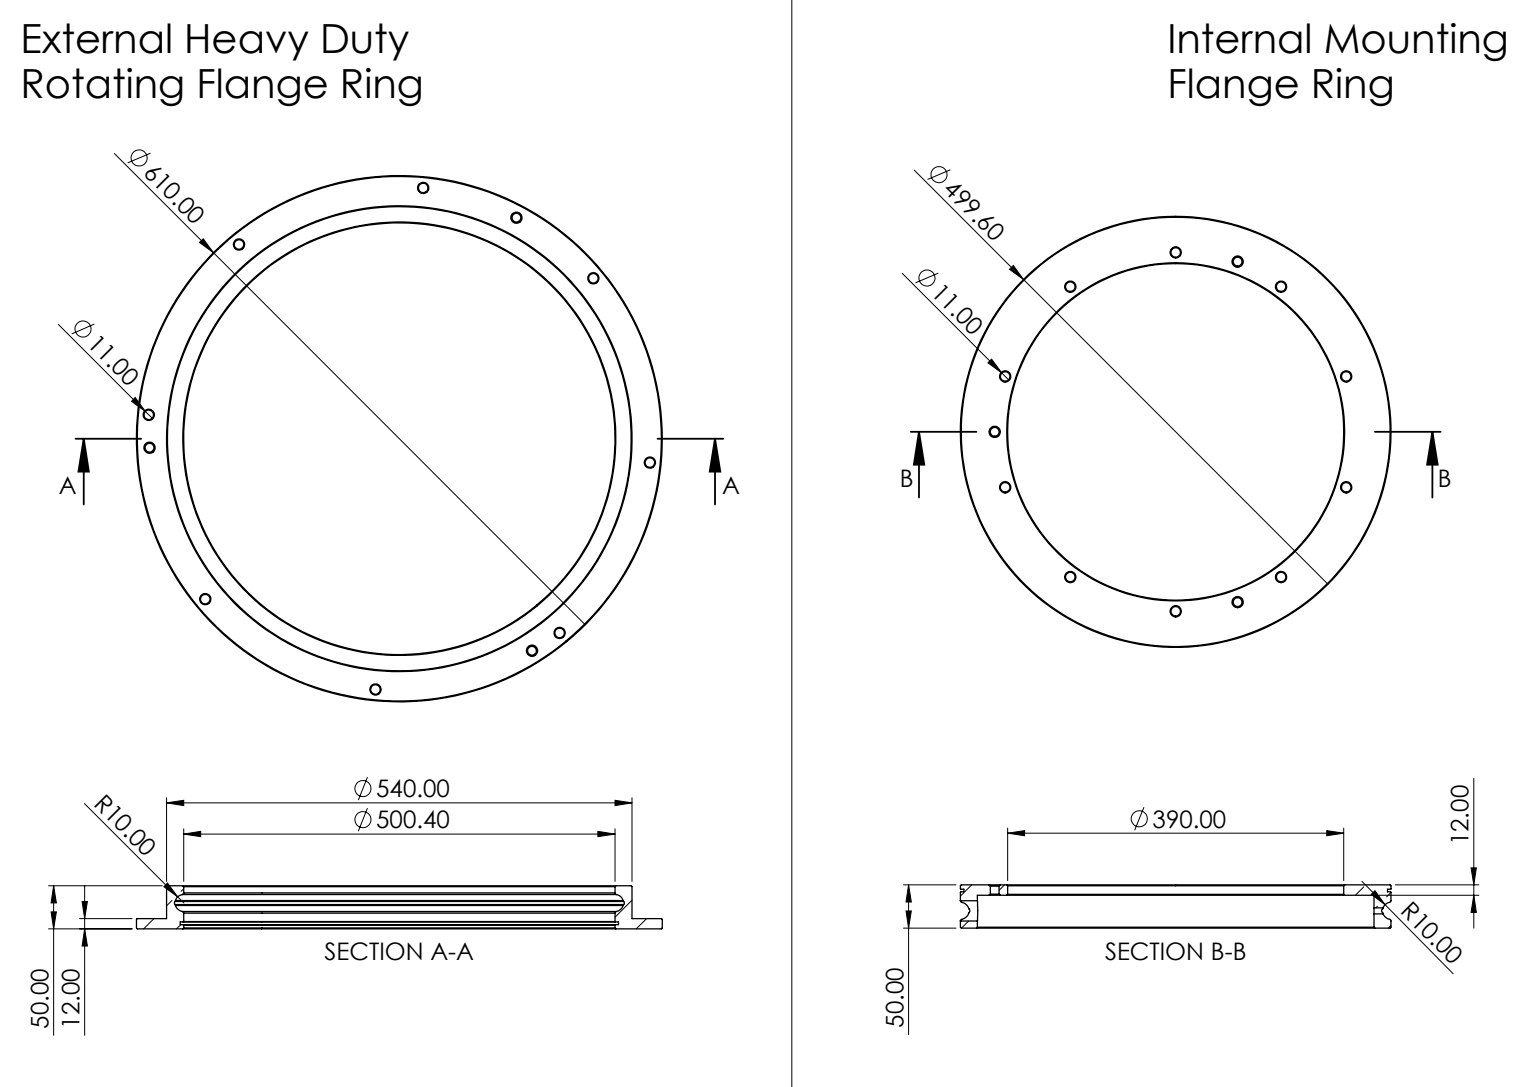
ISO-10303-21;
HEADER;
FILE_DESCRIPTION (('STEP AP214'),
    '1' );
FILE_NAME ('External Heavy Duty Rotating Flange Ring.step',
    '2026-10-09T12:49:55',
    ( '' ),
    ( '' ),
    'SwSTEP 2.0',
    'SolidWorks 2026',
    '' );
FILE_SCHEMA (( 'AUTOMOTIVE_DESIGN' ));
ENDSEC;

DATA;
#2=VECTOR ( 'NONE', #2010, 1000.000000000000000 ) ;
#15=DIRECTION ( 'NONE',  ( 0.6368676505102708330, 0.000000000000000000, 0.7709731485165535192 ) ) ;
#27=ORIENTED_EDGE ( 'NONE', *, *, #7436, .F. ) ;
#31=VECTOR ( 'NONE', #3967, 1000.000000000000000 ) ;
#39=EDGE_CURVE ( 'NONE', #10768, #6987, #12629, .T. ) ;
#40=AXIS2_PLACEMENT_3D ( 'NONE', #6246, #10297, #1175 ) ;
#41=ORIENTED_EDGE ( 'NONE', *, *, #3287, .F. ) ;
#42=EDGE_CURVE ( 'NONE', #9318, #6702, #6889, .T. ) ;
#55=ORIENTED_EDGE ( 'NONE', *, *, #3049, .F. ) ;
#57=CIRCLE ( 'NONE', #1754, 6.500000000000005329 ) ;
#60=CIRCLE ( 'NONE', #11338, 5.499999999999986677 ) ;
#64=DIRECTION ( 'NONE',  ( 0.6368676505102698338, 0.000000000000000000, 0.7709731485165541853 ) ) ;
#65=ORIENTED_EDGE ( 'NONE', *, *, #5983, .T. ) ;
#66=ADVANCED_FACE ( 'NONE', ( #7091 ), #10088, .F. ) ;
#75=CIRCLE ( 'NONE', #5391, 251.1999999999999886 ) ;
#77=AXIS2_PLACEMENT_3D ( 'NONE', #6499, #10557, #9543 ) ;
#79=ORIENTED_EDGE ( 'NONE', *, *, #10538, .F. ) ;
#83=DIRECTION ( 'NONE',  ( -0.000000000000000000, -1.000000000000000000, 0.000000000000000000 ) ) ;
#86=CARTESIAN_POINT ( 'NONE',  ( -182.4625818711933221, -29.00000000000000000, -220.8838070499919297 ) ) ;
#92=EDGE_CURVE ( 'NONE', #10082, #1949, #2942, .T. ) ;
#93=DIRECTION ( 'NONE',  ( 0.000000000000000000, 1.000000000000000000, 0.000000000000000000 ) ) ;
#94=ORIENTED_EDGE ( 'NONE', *, *, #12232, .T. ) ;
#95=ORIENTED_EDGE ( 'NONE', *, *, #11589, .F. ) ;
#96=CONICAL_SURFACE ( 'NONE', #12225, 250.1999999999999602, 0.7853981633975041232 ) ;
#100=CARTESIAN_POINT ( 'NONE',  ( -294.8238222686197787, -18.00000000000000000, -32.70078231947154279 ) ) ;
#104=AXIS2_PLACEMENT_3D ( 'NONE', #9793, #603, #2593 ) ;
#110=ORIENTED_EDGE ( 'NONE', *, *, #7597, .T. ) ;
#112=CIRCLE ( 'NONE', #2851, 5.500000000000007994 ) ;
#113=CARTESIAN_POINT ( 'NONE',  ( 229.2637990951503753, -30.00000000000000000, -180.9540284836414514 ) ) ;
#118=DIRECTION ( 'NONE',  ( -0.000000000000000000, -1.000000000000000000, 0.000000000000000000 ) ) ;
#124=DIRECTION ( 'NONE',  ( -0.6368676505102700558, 0.000000000000000000, -0.7709731485165541853 ) ) ;
#125=AXIS2_PLACEMENT_3D ( 'NONE', #10456, #7067, #12062 ) ;
#128=FACE_OUTER_BOUND ( 'NONE', #4868, .T. ) ;
#140=EDGE_CURVE ( 'NONE', #10237, #12935, #11247, .T. ) ;
#142=CARTESIAN_POINT ( 'NONE',  ( -27.68945685411286561, -30.00000000000000000, 290.6841825403027997 ) ) ;
#148=CARTESIAN_POINT ( 'NONE',  ( -185.9653539489998195, -30.00000000000000000, -225.1241593668329699 ) ) ;
#161=EDGE_CURVE ( 'NONE', #12208, #12419, #5216, .T. ) ;
#169=VERTEX_POINT ( 'NONE', #4404 ) ;
#177=ADVANCED_FACE ( 'NONE', ( #3475, #8488, #10550, #7486, #12547, #4470, #3403, #10415, #12679, #11557, #2351, #9424, #1290 ), #8427, .F. ) ;
#187=DIRECTION ( 'NONE',  ( 0.6368676505102709440, 0.000000000000000000, 0.7709731485165532971 ) ) ;
#195=CARTESIAN_POINT ( 'NONE',  ( -159.9811538081800393, -30.00000000000000000, -193.6684549073582389 ) ) ;
#206=DIRECTION ( 'NONE',  ( 0.6368676505102707219, 0.000000000000000000, 0.7709731485165535192 ) ) ;
#217=AXIS2_PLACEMENT_3D ( 'NONE', #2589, #10592, #3388 ) ;
#222=ORIENTED_EDGE ( 'NONE', *, *, #3793, .T. ) ;
#226=LINE ( 'NONE', #5219, #2394 ) ;
#230=ORIENTED_EDGE ( 'NONE', *, *, #4416, .F. ) ;
#232=ORIENTED_EDGE ( 'NONE', *, *, #7024, .T. ) ;
#233=CARTESIAN_POINT ( 'NONE',  ( 135.8846079354933352, -18.00000000000000000, -256.1940150085812888 ) ) ;
#235=ORIENTED_EDGE ( 'NONE', *, *, #8600, .T. ) ;
#237=VERTEX_POINT ( 'NONE', #3498 ) ;
#239=CARTESIAN_POINT ( 'NONE',  ( -171.9542656377731475, 19.00000000000000000, -208.1627500994694344 ) ) ;
#245=ORIENTED_EDGE ( 'NONE', *, *, #2691, .F. ) ;
#250=DIRECTION ( 'NONE',  ( -0.6368676505102706109, 0.000000000000000000, -0.7709731485165535192 ) ) ;
#251=DIRECTION ( 'NONE',  ( -0.000000000000000000, -1.000000000000000000, 0.000000000000000000 ) ) ;
#253=EDGE_CURVE ( 'NONE', #823, #11992, #3550, .T. ) ;
#266=FACE_OUTER_BOUND ( 'NONE', #2939, .T. ) ;
#268=CONICAL_SURFACE ( 'NONE', #4306, 251.1999999999999886, 0.7853981633974207455 ) ;
#272=CONICAL_SURFACE ( 'NONE', #12608, 6.500000000000005329, 0.7853981633974617127 ) ;
#276=ADVANCED_FACE ( 'NONE', ( #8553 ), #7175, .F. ) ;
#279=CARTESIAN_POINT ( 'NONE',  ( -159.2169126275676945, -3.061616997868385015E-14, -192.7432871291383663 ) ) ;
#282=CARTESIAN_POINT ( 'NONE',  ( 161.8917567597108018, -25.00000000000000000, 195.9813743529078920 ) ) ;
#284=EDGE_LOOP ( 'NONE', ( #11200, #1188, #5610, #7256 ) ) ;
#285=AXIS2_PLACEMENT_3D ( 'NONE', #10507, #6446, #1378 ) ;
#290=CARTESIAN_POINT ( 'NONE',  ( 0.000000000000000000, 2.772967769358929857, 0.000000000000000000 ) ) ;
#291=DIRECTION ( 'NONE',  ( -0.000000000000000000, -1.000000000000000000, 0.000000000000000000 ) ) ;
#294=CIRCLE ( 'NONE', #504, 5.500000000000015099 ) ;
#318=DIRECTION ( 'NONE',  ( 0.6368676505102716101, 0.000000000000000000, 0.7709731485165527420 ) ) ;
#321=DIRECTION ( 'NONE',  ( 0.000000000000000000, 1.000000000000000000, 0.000000000000000000 ) ) ;
#322=ORIENTED_EDGE ( 'NONE', *, *, #332, .F. ) ;
#327=VERTEX_POINT ( 'NONE', #7610 ) ;
#332=EDGE_CURVE ( 'NONE', #5214, #8298, #11654, .T. ) ;
#352=CARTESIAN_POINT ( 'NONE',  ( -171.9542656377731475, -18.00000000000000000, -208.1627500994694344 ) ) ;
#353=EDGE_LOOP ( 'NONE', ( #11784, #3307 ) ) ;
#354=VERTEX_POINT ( 'NONE', #3337 ) ;
#355=EDGE_CURVE ( 'NONE', #8227, #8752, #1859, .T. ) ;
#357=CARTESIAN_POINT ( 'NONE',  ( 235.1468102975488250, -18.00000000000000000, -194.2446334056325554 ) ) ;
#366=VERTEX_POINT ( 'NONE', #1547 ) ;
#367=DIRECTION ( 'NONE',  ( -0.6368676505102707219, 0.000000000000000000, -0.7709731485165535192 ) ) ;
#372=LINE ( 'NONE', #9371, #6679 ) ;
#373=CARTESIAN_POINT ( 'NONE',  ( 221.6213872890270977, -19.00000000000000000, -190.2057062658400923 ) ) ;
#377=CYLINDRICAL_SURFACE ( 'NONE', #4954, 5.100000000000003197 ) ;
#380=DIRECTION ( 'NONE',  ( -0.000000000000000000, -1.000000000000000000, 0.000000000000000000 ) ) ;
#383=DIRECTION ( 'NONE',  ( 0.6368676505102707219, 0.000000000000000000, 0.7709731485165536302 ) ) ;
#385=ADVANCED_FACE ( 'NONE', ( #12734 ), #10286, .F. ) ;
#392=CARTESIAN_POINT ( 'NONE',  ( -166.5596220099214690, -3.327561323230905366, -201.6321540179175713 ) ) ;
#401=ORIENTED_EDGE ( 'NONE', *, *, #140, .T. ) ;
#403=DIRECTION ( 'NONE',  ( 0.7709731485165535192, -0.000000000000000000, -0.6368676505102707219 ) ) ;
#410=DIRECTION ( 'NONE',  ( 0.6368676505102707219, 0.000000000000000000, 0.7709731485165535192 ) ) ;
#413=AXIS2_PLACEMENT_3D ( 'NONE', #9466, #8658, #6404 ) ;
#415=EDGE_LOOP ( 'NONE', ( #4979, #4482 ) ) ;
#418=ADVANCED_FACE ( 'NONE', ( #10744, #4871, #681, #11821, #9730, #1615, #2543, #12876, #6620, #1747, #10675, #555, #13009 ), #3605, .F. ) ;
#419=VECTOR ( 'NONE', #10160, 1000.000000000000000 ) ;
#424=FACE_OUTER_BOUND ( 'NONE', #2937, .T. ) ;
#427=CARTESIAN_POINT ( 'NONE',  ( -286.5445428119863323, -30.00000000000000000, -22.67813138875635204 ) ) ;
#435=DIRECTION ( 'NONE',  ( -0.000000000000000000, -1.000000000000000000, 0.000000000000000000 ) ) ;
#438=CARTESIAN_POINT ( 'NONE',  ( 171.9542656377731191, 19.00000000000000000, 208.1627500994694628 ) ) ;
#445=ADVANCED_FACE ( 'NONE', ( #12807 ), #6891, .F. ) ;
#446=EDGE_CURVE ( 'NONE', #12435, #9116, #11362, .T. ) ;
#449=ORIENTED_EDGE ( 'NONE', *, *, #355, .T. ) ;
#450=DIRECTION ( 'NONE',  ( 0.000000000000000000, 1.000000000000000000, 0.000000000000000000 ) ) ;
#452=CARTESIAN_POINT ( 'NONE',  ( -31.19222893191933821, -29.00000000000000000, 286.4438302234618163 ) ) ;
#454=CARTESIAN_POINT ( 'NONE',  ( 182.4625818711949137, -29.00000000000000000, 220.8838070499906507 ) ) ;
#455=PLANE ( 'NONE',  #2846 ) ;
#461=DIRECTION ( 'NONE',  ( 0.4503334343941581830, -0.7071067811865450192, 0.5451603414288000993 ) ) ;
#471=FACE_OUTER_BOUND ( 'NONE', #1035, .T. ) ;
#472=APPLICATION_CONTEXT ( 'automotive_design' ) ;
#481=AXIS2_PLACEMENT_3D ( 'NONE', #1897, #9541, #12361 ) ;
#484=AXIS2_PLACEMENT_3D ( 'NONE', #2681, #9957, #3755 ) ;
#500=DIRECTION ( 'NONE',  ( -0.6368676505102737195, 0.000000000000000000, -0.7709731485165509657 ) ) ;
#504=AXIS2_PLACEMENT_3D ( 'NONE', #4431, #380, #12767 ) ;
#507=DIRECTION ( 'NONE',  ( -0.000000000000000000, -1.000000000000000000, 0.000000000000000000 ) ) ;
#509=CARTESIAN_POINT ( 'NONE',  ( 185.9653539490014111, -30.00000000000000000, 225.1241593668316625 ) ) ;
#511=FACE_OUTER_BOUND ( 'NONE', #4843, .T. ) ;
#512=EDGE_CURVE ( 'NONE', #4498, #11239, #1570, .T. ) ;
#514=ORIENTED_EDGE ( 'NONE', *, *, #864, .T. ) ;
#518=CARTESIAN_POINT ( 'NONE',  ( 159.3442861576696998, -25.50000000000000000, 192.8974817588417352 ) ) ;
#526=DIRECTION ( 'NONE',  ( -0.6368676505102698338, 0.000000000000000000, -0.7709731485165541853 ) ) ;
#531=ORIENTED_EDGE ( 'NONE', *, *, #1101, .F. ) ;
#535=EDGE_CURVE ( 'NONE', #8515, #6953, #11631, .T. ) ;
#538=CARTESIAN_POINT ( 'NONE',  ( -290.6841825403030839, -19.00000000000000000, -27.68945685411394919 ) ) ;
#539=CARTESIAN_POINT ( 'NONE',  ( 27.68945685411497593, -19.00000000000000000, -290.6841825403026291 ) ) ;
#549=AXIS2_PLACEMENT_3D ( 'NONE', #4500, #3705, #6585 ) ;
#555=FACE_BOUND ( 'NONE', #1673, .T. ) ;
#557=CIRCLE ( 'NONE', #5230, 250.7000000000000171 ) ;
#558=DIRECTION ( 'NONE',  ( 0.6368676505102737195, 0.000000000000000000, 0.7709731485165509657 ) ) ;
#561=CARTESIAN_POINT ( 'NONE',  ( 182.4625818711949137, -19.00000000000000000, 220.8838070499906223 ) ) ;
#562=ORIENTED_EDGE ( 'NONE', *, *, #6556, .F. ) ;
#564=VERTEX_POINT ( 'NONE', #6140 ) ;
#565=CYLINDRICAL_SURFACE ( 'NONE', #12328, 254.1999999999999886 ) ;
#566=ORIENTED_EDGE ( 'NONE', *, *, #6725, .F. ) ;
#567=ORIENTED_EDGE ( 'NONE', *, *, #4107, .F. ) ;
#571=DIRECTION ( 'NONE',  ( -0.000000000000000000, -1.000000000000000000, 0.000000000000000000 ) ) ;
#577=ORIENTED_EDGE ( 'NONE', *, *, #3546, .T. ) ;
#581=DIRECTION ( 'NONE',  ( -0.000000000000000000, -1.000000000000000000, 0.000000000000000000 ) ) ;
#591=CARTESIAN_POINT ( 'NONE',  ( -0.000000000000000000, -3.165711975795909891E-14, 0.000000000000000000 ) ) ;
#592=ORIENTED_EDGE ( 'NONE', *, *, #10942, .T. ) ;
#598=DIRECTION ( 'NONE',  ( -0.000000000000000000, -1.000000000000000000, 0.000000000000000000 ) ) ;
#599=CARTESIAN_POINT ( 'NONE',  ( -0.000000000000000000, -11.79660968244695951, 0.000000000000000000 ) ) ;
#600=DIRECTION ( 'NONE',  ( -0.000000000000000000, -1.000000000000000000, 0.000000000000000000 ) ) ;
#603=DIRECTION ( 'NONE',  ( -0.000000000000000000, -1.000000000000000000, 0.000000000000000000 ) ) ;
#604=AXIS2_PLACEMENT_3D ( 'NONE', #8620, #4664, #3604 ) ;
#607=EDGE_CURVE ( 'NONE', #4062, #10624, #1004, .T. ) ;
#613=DIRECTION ( 'NONE',  ( -0.7709731485165535192, 0.000000000000000000, 0.6368676505102708330 ) ) ;
#614=AXIS2_PLACEMENT_3D ( 'NONE', #8258, #6261, #383 ) ;
#616=VECTOR ( 'NONE', #8753, 1000.000000000000000 ) ;
#619=DIRECTION ( 'NONE',  ( -0.6368676505102706109, 0.000000000000000000, -0.7709731485165535192 ) ) ;
#626=AXIS2_PLACEMENT_3D ( 'NONE', #7112, #7979, #4970 ) ;
#631=ORIENTED_EDGE ( 'NONE', *, *, #8325, .T. ) ;
#633=CARTESIAN_POINT ( 'NONE',  ( 140.0242476638101152, -30.00000000000000000, -251.1826895432237166 ) ) ;
#637=CARTESIAN_POINT ( 'NONE',  ( -27.68945685411286561, -30.00000000000000000, 290.6841825403027997 ) ) ;
#639=CIRCLE ( 'NONE', #9812, 5.100000000000003197 ) ;
#648=DIRECTION ( 'NONE',  ( 0.6368676505102716101, 0.000000000000000000, 0.7709731485165527420 ) ) ;
#656=DIRECTION ( 'NONE',  ( -0.4503334343941582940, -0.7071067811865450192, -0.5451603414288000993 ) ) ;
#660=ORIENTED_EDGE ( 'NONE', *, *, #9431, .T. ) ;
#663=EDGE_LOOP ( 'NONE', ( #7219, #7167, #8642, #12298 ) ) ;
#666=DIRECTION ( 'NONE',  ( -0.4503334343941627904, -0.7071067811865381358, -0.5451603414288054283 ) ) ;
#667=CARTESIAN_POINT ( 'NONE',  ( -287.1814104624966149, -19.00000000000000000, -23.44910453727290189 ) ) ;
#668=CARTESIAN_POINT ( 'NONE',  ( 0.000000000000000000, 0.000000000000000000, 0.000000000000000000 ) ) ;
#670=CARTESIAN_POINT ( 'NONE',  ( -229.2637990951503753, -18.00000000000000000, 180.9540284836414514 ) ) ;
#673=VECTOR ( 'NONE', #3157, 1000.000000000000000 ) ;
#676=ORIENTED_EDGE ( 'NONE', *, *, #6226, .T. ) ;
#679=ORIENTED_EDGE ( 'NONE', *, *, #4416, .T. ) ;
#681=FACE_BOUND ( 'NONE', #2232, .T. ) ;
#685=DIRECTION ( 'NONE',  ( 0.000000000000000000, 1.000000000000000000, 0.000000000000000000 ) ) ;
#688=AXIS2_PLACEMENT_3D ( 'NONE', #9443, #1239, #11509 ) ;
#689=CARTESIAN_POINT ( 'NONE',  ( -290.6841825403030839, -30.00000000000000000, -27.68945685411394919 ) ) ;
#695=EDGE_LOOP ( 'NONE', ( #12036, #7828, #9009, #10772 ) ) ;
#702=ADVANCED_FACE ( 'NONE', ( #4135 ), #8217, .F. ) ;
#706=LINE ( 'NONE', #8639, #7975 ) ;
#708=EDGE_CURVE ( 'NONE', #3236, #5526, #10611, .T. ) ;
#710=CARTESIAN_POINT ( 'NONE',  ( -27.68945685411286561, -19.00000000000000000, 290.6841825403027997 ) ) ;
#711=VECTOR ( 'NONE', #2929, 1000.000000000000000 ) ;
#712=ORIENTED_EDGE ( 'NONE', *, *, #12259, .T. ) ;
#715=ORIENTED_EDGE ( 'NONE', *, *, #5260, .T. ) ;
#718=CARTESIAN_POINT ( 'NONE',  ( 31.82909658243173467, -30.00000000000000000, -285.6728570749450569 ) ) ;
#720=AXIS2_PLACEMENT_3D ( 'NONE', #12565, #1304, #3418 ) ;
#727=ORIENTED_EDGE ( 'NONE', *, *, #5095, .T. ) ;
#736=FACE_OUTER_BOUND ( 'NONE', #11166, .T. ) ;
#741=AXIS2_PLACEMENT_3D ( 'NONE', #10234, #5164, #9243 ) ;
#750=ORIENTED_EDGE ( 'NONE', *, *, #4772, .F. ) ;
#752=CARTESIAN_POINT ( 'NONE',  ( -0.000000000000000000, -21.50000000000000000, 0.000000000000000000 ) ) ;
#753=CARTESIAN_POINT ( 'NONE',  ( -0.000000000000000000, -18.00000000000000000, 0.000000000000000000 ) ) ;
#757=CARTESIAN_POINT ( 'NONE',  ( 0.000000000000000000, 20.00000000000000000, 0.000000000000000000 ) ) ;
#761=COLOUR_RGB ( '', 0.72549020, 0.75294118, 0.79215686) ;
#764=CARTESIAN_POINT ( 'NONE',  ( 24.18668477630849267, -19.00000000000000000, -294.9245348571437262 ) ) ;
#767=CARTESIAN_POINT ( 'NONE',  ( -181.8257142206830679, -30.00000000000000000, -220.1128339014753692 ) ) ;
#779=VERTEX_POINT ( 'NONE', #9336 ) ;
#795=FACE_OUTER_BOUND ( 'NONE', #836, .T. ) ;
#805=AXIS2_PLACEMENT_3D ( 'NONE', #6711, #10765, #10635 ) ;
#814=DIRECTION ( 'NONE',  ( -0.000000000000000000, -1.000000000000000000, 0.000000000000000000 ) ) ;
#815=ORIENTED_EDGE ( 'NONE', *, *, #7409, .F. ) ;
#823=VERTEX_POINT ( 'NONE', #2331 ) ;
#830=DIRECTION ( 'NONE',  ( 0.6368676505102708330, 0.000000000000000000, 0.7709731485165535192 ) ) ;
#833=CARTESIAN_POINT ( 'NONE',  ( 0.000000000000000000, 20.00000000000000000, 0.000000000000000000 ) ) ;
#836=EDGE_LOOP ( 'NONE', ( #6634, #7940, #7084, #12038 ) ) ;
#837=FACE_OUTER_BOUND ( 'NONE', #10019, .T. ) ;
#855=CONICAL_SURFACE ( 'NONE', #12555, 6.500000000000005329, 0.7853981633974476129 ) ;
#856=ORIENTED_EDGE ( 'NONE', *, *, #12058, .F. ) ;
#857=ORIENTED_EDGE ( 'NONE', *, *, #9638, .T. ) ;
#859=ORIENTED_EDGE ( 'NONE', *, *, #3793, .F. ) ;
#862=CARTESIAN_POINT ( 'NONE',  ( -0.000000000000000000, -29.00000000000000000, 0.000000000000000000 ) ) ;
#864=EDGE_CURVE ( 'NONE', #6987, #11199, #7273, .T. ) ;
#873=ORIENTED_EDGE ( 'NONE', *, *, #8104, .T. ) ;
#877=CARTESIAN_POINT ( 'NONE',  ( -290.6841825403030839, -18.00000000000000000, -27.68945685411394919 ) ) ;
#886=ORIENTED_EDGE ( 'NONE', *, *, #7689, .F. ) ;
#890=ORIENTED_EDGE ( 'NONE', *, *, #10293, .T. ) ;
#891=DIRECTION ( 'NONE',  ( 0.6368676505102707219, 0.000000000000000000, 0.7709731485165535192 ) ) ;
#893=CARTESIAN_POINT ( 'NONE',  ( 160.6180214586902366, 11.79660968244693997, 194.4394280558747994 ) ) ;
#894=AXIS2_PLACEMENT_3D ( 'NONE', #1605, #600, #9791 ) ;
#895=EDGE_CURVE ( 'NONE', #6702, #6924, #4337, .T. ) ;
#900=VERTEX_POINT ( 'NONE', #8538 ) ;
#908=LINE ( 'NONE', #2961, #1944 ) ;
#910=DIRECTION ( 'NONE',  ( 0.6368676505102709440, 0.000000000000000000, 0.7709731485165532971 ) ) ;
#911=EDGE_CURVE ( 'NONE', #10031, #1416, #5411, .T. ) ;
#914=APPLICATION_CONTEXT ( 'automotive_design' ) ;
#919=UNCERTAINTY_MEASURE_WITH_UNIT (LENGTH_MEASURE( 1.000000000000000082E-05 ), #5049, 'distance_accuracy_value', 'NONE');
#920=ORIENTED_EDGE ( 'NONE', *, *, #11171, .T. ) ;
#927=VECTOR ( 'NONE', #6570, 1000.000000000000000 ) ;
#931=DIRECTION ( 'NONE',  ( 0.6368676505102707219, 0.000000000000000000, 0.7709731485165535192 ) ) ;
#935=SURFACE_STYLE_USAGE ( .BOTH. , #10063 ) ;
#941=VERTEX_POINT ( 'NONE', #11733 ) ;
#943=CARTESIAN_POINT ( 'NONE',  ( 286.5445428119865028, -30.00000000000000000, 22.67813138875427015 ) ) ;
#945=VECTOR ( 'NONE', #7892, 1000.000000000000000 ) ;
#949=DIRECTION ( 'NONE',  ( -0.000000000000000000, -1.000000000000000000, 0.000000000000000000 ) ) ;
#955=AXIS2_PLACEMENT_3D ( 'NONE', #9704, #11726, #9580 ) ;
#957=CARTESIAN_POINT ( 'NONE',  ( -289.8128292627096130, -30.00000000000000000, 10.41748504886635907 ) ) ;
#958=EDGE_LOOP ( 'NONE', ( #8262, #10296, #3960, #7089 ) ) ;
#959=ORIENTED_EDGE ( 'NONE', *, *, #1758, .F. ) ;
#960=CARTESIAN_POINT ( 'NONE',  ( -0.000000000000000000, -11.79660968244695951, 0.000000000000000000 ) ) ;
#965=DIRECTION ( 'NONE',  ( 0.4503334343941555740, 0.7071067811865490160, 0.5451603414287971017 ) ) ;
#969=ORIENTED_EDGE ( 'NONE', *, *, #5981, .F. ) ;
#971=ORIENTED_EDGE ( 'NONE', *, *, #6486, .F. ) ;
#975=DIRECTION ( 'NONE',  ( -0.6368676505102707219, 0.000000000000000000, -0.7709731485165535192 ) ) ;
#984=ORIENTED_EDGE ( 'NONE', *, *, #6119, .T. ) ;
#986=EDGE_CURVE ( 'NONE', #7844, #5825, #4648, .T. ) ;
#989=ORIENTED_EDGE ( 'NONE', *, *, #7409, .T. ) ;
#996=SURFACE_STYLE_FILL_AREA ( #11127 ) ;
#1004=LINE ( 'NONE', #4497, #7838 ) ;
#1005=PLANE ( 'NONE',  #8520 ) ;
#1018=ORIENTED_EDGE ( 'NONE', *, *, #10942, .F. ) ;
#1019=DIRECTION ( 'NONE',  ( 0.6368676505102707219, 0.000000000000000000, 0.7709731485165535192 ) ) ;
#1023=EDGE_CURVE ( 'NONE', #11697, #2079, #4230, .T. ) ;
#1027=ORIENTED_EDGE ( 'NONE', *, *, #1507, .T. ) ;
#1029=TOROIDAL_SURFACE ( 'NONE', #4427, 252.1999999999999886, 2.000000000000000000 ) ;
#1033=ORIENTED_EDGE ( 'NONE', *, *, #11937, .T. ) ;
#1035=EDGE_LOOP ( 'NONE', ( #566, #11162, #7813, #5039 ) ) ;
#1043=VECTOR ( 'NONE', #4814, 1000.000000000000000 ) ;
#1047=CIRCLE ( 'NONE', #6376, 251.1999999999999886 ) ;
#1061=CIRCLE ( 'NONE', #12129, 5.100000000000003197 ) ;
#1067=ORIENTED_EDGE ( 'NONE', *, *, #11182, .T. ) ;
#1075=CYLINDRICAL_SURFACE ( 'NONE', #11982, 5.500000000000007994 ) ;
#1077=VECTOR ( 'NONE', #1474, 1000.000000000000000 ) ;
#1079=ORIENTED_EDGE ( 'NONE', *, *, #1023, .T. ) ;
#1086=ADVANCED_FACE ( 'NONE', ( #736 ), #6375, .F. ) ;
#1092=DIRECTION ( 'NONE',  ( 0.6368676505102707219, 0.000000000000000000, 0.7709731485165535192 ) ) ;
#1095=ORIENTED_EDGE ( 'NONE', *, *, #10168, .F. ) ;
#1096=DIRECTION ( 'NONE',  ( -0.6368676505102707219, 0.000000000000000000, -0.7709731485165535192 ) ) ;
#1100=VERTEX_POINT ( 'NONE', #2649 ) ;
#1101=EDGE_CURVE ( 'NONE', #10423, #5861, #4770, .T. ) ;
#1102=CARTESIAN_POINT ( 'NONE',  ( 225.1241593668336236, -30.00000000000000000, -185.9653539489990521 ) ) ;
#1105=CARTESIAN_POINT ( 'NONE',  ( -0.000000000000000000, -3.165711975795909891E-14, 0.000000000000000000 ) ) ;
#1107=DIRECTION ( 'NONE',  ( -0.000000000000000000, -1.000000000000000000, 0.000000000000000000 ) ) ;
#1108=DIRECTION ( 'NONE',  ( 0.6368676505102716101, 0.000000000000000000, 0.7709731485165527420 ) ) ;
#1109=ADVANCED_FACE ( 'NONE', ( #9059 ), #7125, .T. ) ;
#1114=ORIENTED_EDGE ( 'NONE', *, *, #42, .T. ) ;
#1115=DIRECTION ( 'NONE',  ( -0.000000000000000000, -1.000000000000000000, 0.000000000000000000 ) ) ;
#1119=FACE_OUTER_BOUND ( 'NONE', #12151, .T. ) ;
#1125=CARTESIAN_POINT ( 'NONE',  ( 185.9653539490014111, -19.00000000000000000, 225.1241593668316625 ) ) ;
#1127=AXIS2_PLACEMENT_3D ( 'NONE', #9176, #12175, #4106 ) ;
#1133=DIRECTION ( 'NONE',  ( 0.000000000000000000, 1.000000000000000000, 0.000000000000000000 ) ) ;
#1135=ORIENTED_EDGE ( 'NONE', *, *, #3577, .F. ) ;
#1137=ADVANCED_FACE ( 'NONE', ( #5929 ), #1377, .T. ) ;
#1144=VECTOR ( 'NONE', #5770, 1000.000000000000000 ) ;
#1154=ADVANCED_FACE ( 'NONE', ( #795 ), #2947, .T. ) ;
#1155=ORIENTED_EDGE ( 'NONE', *, *, #12673, .T. ) ;
#1156=EDGE_CURVE ( 'NONE', #12208, #9851, #8613, .T. ) ;
#1159=DIRECTION ( 'NONE',  ( -0.000000000000000000, -1.000000000000000000, 0.000000000000000000 ) ) ;
#1166=AXIS2_PLACEMENT_3D ( 'NONE', #11964, #2622, #4559 ) ;
#1170=VERTEX_POINT ( 'NONE', #8929 ) ;
#1175=DIRECTION ( 'NONE',  ( 0.6368676505102707219, 0.000000000000000000, 0.7709731485165535192 ) ) ;
#1187=CIRCLE ( 'NONE', #8225, 6.500000000000005329 ) ;
#1188=ORIENTED_EDGE ( 'NONE', *, *, #8602, .F. ) ;
#1189=VECTOR ( 'NONE', #11301, 1000.000000000000000 ) ;
#1193=ORIENTED_EDGE ( 'NONE', *, *, #6647, .T. ) ;
#1196=DIRECTION ( 'NONE',  ( 0.6368676505102707219, 0.000000000000000000, 0.7709731485165535192 ) ) ;
#1199=ADVANCED_FACE ( 'NONE', ( #6721 ), #10305, .F. ) ;
#1200=DIRECTION ( 'NONE',  ( 0.000000000000000000, 1.000000000000000000, 0.000000000000000000 ) ) ;
#1203=CARTESIAN_POINT ( 'NONE',  ( -289.8128292627096130, -19.40000000000000213, 10.41748504886635907 ) ) ;
#1208=FACE_OUTER_BOUND ( 'NONE', #353, .T. ) ;
#1216=DIRECTION ( 'NONE',  ( 0.000000000000000000, 1.000000000000000000, 0.000000000000000000 ) ) ;
#1221=DIRECTION ( 'NONE',  ( 0.6368676505102708330, 0.000000000000000000, 0.7709731485165535192 ) ) ;
#1224=CARTESIAN_POINT ( 'NONE',  ( -229.2637990951503753, -30.00000000000000000, 180.9540284836414514 ) ) ;
#1228=ADVANCED_FACE ( 'NONE', ( #7706, #1712 ), #455, .F. ) ;
#1231=ORIENTED_EDGE ( 'NONE', *, *, #3028, .T. ) ;
#1233=ORIENTED_EDGE ( 'NONE', *, *, #8587, .T. ) ;
#1234=ORIENTED_EDGE ( 'NONE', *, *, #895, .T. ) ;
#1236=CARTESIAN_POINT ( 'NONE',  ( -0.000000000000000000, -1.848645179577135034, 0.000000000000000000 ) ) ;
#1238=CARTESIAN_POINT ( 'NONE',  ( -225.1241593668336236, -18.00000000000000000, 185.9653539489990521 ) ) ;
#1239=DIRECTION ( 'NONE',  ( -0.000000000000000000, -1.000000000000000000, 0.000000000000000000 ) ) ;
#1240=CARTESIAN_POINT ( 'NONE',  ( 0.000000000000000000, 0.000000000000000000, 0.000000000000000000 ) ) ;
#1244=VERTEX_POINT ( 'NONE', #718 ) ;
#1247=DIRECTION ( 'NONE',  ( -0.000000000000000000, -1.000000000000000000, 0.000000000000000000 ) ) ;
#1250=ORIENTED_EDGE ( 'NONE', *, *, #5677, .T. ) ;
#1251=AXIS2_PLACEMENT_3D ( 'NONE', #9452, #3363, #11450 ) ;
#1252=EDGE_CURVE ( 'NONE', #10483, #10082, #3490, .T. ) ;
#1255=ADVANCED_FACE ( 'NONE', ( #10775 ), #11745, .F. ) ;
#1258=AXIS2_PLACEMENT_3D ( 'NONE', #12752, #3616, #7684 ) ;
#1265=AXIS2_PLACEMENT_3D ( 'NONE', #8906, #12976, #4769 ) ;
#1268=ORIENTED_EDGE ( 'NONE', *, *, #8533, .T. ) ;
#1272=DIRECTION ( 'NONE',  ( -0.4503334343941627904, -0.7071067811865381358, -0.5451603414288054283 ) ) ;
#1273=VECTOR ( 'NONE', #5631, 1000.000000000000000 ) ;
#1274=CARTESIAN_POINT ( 'NONE',  ( -289.8128292627096130, -30.00000000000000000, 10.41748504886635907 ) ) ;
#1280=CARTESIAN_POINT ( 'NONE',  ( 228.6269314446401211, -19.00000000000000000, -181.7250016321579835 ) ) ;
#1287=ORIENTED_EDGE ( 'NONE', *, *, #512, .T. ) ;
#1290=FACE_OUTER_BOUND ( 'NONE', #10006, .T. ) ;
#1293=DIRECTION ( 'NONE',  ( -0.6368676505102707219, 0.000000000000000000, -0.7709731485165536302 ) ) ;
#1300=FACE_OUTER_BOUND ( 'NONE', #2873, .T. ) ;
#1301=EDGE_LOOP ( 'NONE', ( #12296, #7141, #10815, #12253 ) ) ;
#1303=EDGE_CURVE ( 'NONE', #5861, #10423, #3419, .T. ) ;
#1304=DIRECTION ( 'NONE',  ( -0.000000000000000000, -1.000000000000000000, 0.000000000000000000 ) ) ;
#1307=CARTESIAN_POINT ( 'NONE',  ( -225.1241593668336236, -30.00000000000000000, 185.9653539489990521 ) ) ;
#1312=ORIENTED_EDGE ( 'NONE', *, *, #4894, .T. ) ;
#1314=CARTESIAN_POINT ( 'NONE',  ( 153.9282213272189495, -28.60000000000000142, 245.7765299597151341 ) ) ;
#1318=LINE ( 'NONE', #4501, #9779 ) ;
#1321=EDGE_CURVE ( 'NONE', #1858, #4661, #11845, .T. ) ;
#1325=CARTESIAN_POINT ( 'NONE',  ( 158.0678610555357295, -30.00000000000000000, 250.7878554250727632 ) ) ;
#1327=CARTESIAN_POINT ( 'NONE',  ( 0.000000000000000000, 20.00000000000000000, 0.000000000000000000 ) ) ;
#1333=EDGE_LOOP ( 'NONE', ( #4898, #4678 ) ) ;
#1342=CIRCLE ( 'NONE', #9629, 10.00000000000000178 ) ;
#1346=ADVANCED_FACE ( 'NONE', ( #6589 ), #8973, .F. ) ;
#1347=EDGE_LOOP ( 'NONE', ( #9668, #11883, #1234, #3830 ) ) ;
#1348=CIRCLE ( 'NONE', #1127, 10.00000000000000178 ) ;
#1352=ORIENTED_EDGE ( 'NONE', *, *, #7689, .T. ) ;
#1359=CARTESIAN_POINT ( 'NONE',  ( 153.9282213272189495, -30.00000000000000000, 245.7765299597151341 ) ) ;
#1372=CARTESIAN_POINT ( 'NONE',  ( 158.0678610555357295, -30.00000000000000000, 250.7878554250727632 ) ) ;
#1377=TOROIDAL_SURFACE ( 'NONE', #12236, 261.5294117647060261, 2.000000000000000000 ) ;
#1378=DIRECTION ( 'NONE',  ( -0.6368676505102698338, 0.000000000000000000, -0.7709731485165542964 ) ) ;
#1381=CARTESIAN_POINT ( 'NONE',  ( 185.9653539490014111, -30.00000000000000000, 225.1241593668316625 ) ) ;
#1384=CARTESIAN_POINT ( 'NONE',  ( 0.000000000000000000, 19.00000000000000000, 0.000000000000000000 ) ) ;
#1398=ADVANCED_FACE ( 'NONE', ( #1640 ), #3211, .F. ) ;
#1402=VECTOR ( 'NONE', #5824, 1000.000000000000114 ) ;
#1405=CYLINDRICAL_SURFACE ( 'NONE', #6256, 5.500000000000007994 ) ;
#1409=DIRECTION ( 'NONE',  ( -0.000000000000000000, -1.000000000000000000, 0.000000000000000000 ) ) ;
#1413=DIRECTION ( 'NONE',  ( -0.000000000000000000, -1.000000000000000000, 0.000000000000000000 ) ) ;
#1415=ORIENTED_EDGE ( 'NONE', *, *, #3005, .F. ) ;
#1416=VERTEX_POINT ( 'NONE', #11976 ) ;
#1429=AXIS2_PLACEMENT_3D ( 'NONE', #12612, #4348, #11623 ) ;
#1433=DIRECTION ( 'NONE',  ( -0.000000000000000000, -1.000000000000000000, 0.000000000000000000 ) ) ;
#1434=EDGE_CURVE ( 'NONE', #5762, #8072, #10667, .T. ) ;
#1437=CYLINDRICAL_SURFACE ( 'NONE', #7753, 270.0000000000000000 ) ;
#1447=DIRECTION ( 'NONE',  ( -0.000000000000000000, -1.000000000000000000, 0.000000000000000000 ) ) ;
#1452=DIRECTION ( 'NONE',  ( 0.6368676505102689456, 0.000000000000000000, 0.7709731485165549625 ) ) ;
#1456=AXIS2_PLACEMENT_3D ( 'NONE', #5382, #2248, #10445 ) ;
#1457=CONICAL_SURFACE ( 'NONE', #6578, 5.500000000000015099, 0.7853981633974461696 ) ;
#1461=AXIS2_PLACEMENT_3D ( 'NONE', #10142, #7221, #4277 ) ;
#1465=CARTESIAN_POINT ( 'NONE',  ( 225.1241593668336236, -30.00000000000000000, -185.9653539489990521 ) ) ;
#1474=DIRECTION ( 'NONE',  ( -0.000000000000000000, -1.000000000000000000, 0.000000000000000000 ) ) ;
#1494=ADVANCED_FACE ( 'NONE', ( #2962 ), #8547, .F. ) ;
#1495=CARTESIAN_POINT ( 'NONE',  ( -23.54981712579610331, -30.00000000000000000, 295.6955080056604288 ) ) ;
#1496=EDGE_LOOP ( 'NONE', ( #3668, #5704 ) ) ;
#1499=DIRECTION ( 'NONE',  ( -0.000000000000000000, -1.000000000000000000, 0.000000000000000000 ) ) ;
#1506=DIRECTION ( 'NONE',  ( 0.6368676505102716101, 0.000000000000000000, 0.7709731485165527420 ) ) ;
#1507=EDGE_CURVE ( 'NONE', #10768, #8072, #5850, .T. ) ;
#1516=DIRECTION ( 'NONE',  ( 0.000000000000000000, 1.000000000000000000, 0.000000000000000000 ) ) ;
#1520=AXIS2_PLACEMENT_3D ( 'NONE', #2880, #9030, #4018 ) ;
#1521=DIRECTION ( 'NONE',  ( 0.7709731485165535192, 0.000000000000000000, -0.6368676505102707219 ) ) ;
#1524=EDGE_CURVE ( 'NONE', #8945, #4077, #11104, .T. ) ;
#1526=ORIENTED_EDGE ( 'NONE', *, *, #4011, .F. ) ;
#1534=DIRECTION ( 'NONE',  ( 0.6368676505102707219, 0.000000000000000000, 0.7709731485165535192 ) ) ;
#1536=DIRECTION ( 'NONE',  ( -0.000000000000000000, -1.000000000000000000, 0.000000000000000000 ) ) ;
#1540=VECTOR ( 'NONE', #7162, 1000.000000000000000 ) ;
#1547=CARTESIAN_POINT ( 'NONE',  ( 171.3173979872628365, 20.00000000000000000, 207.3917769509529307 ) ) ;
#1555=DIRECTION ( 'NONE',  ( 0.000000000000000000, 1.000000000000000000, 0.000000000000000000 ) ) ;
#1561=FACE_OUTER_BOUND ( 'NONE', #6989, .T. ) ;
#1563=ORIENTED_EDGE ( 'NONE', *, *, #7436, .T. ) ;
#1569=CARTESIAN_POINT ( 'NONE',  ( -159.9811538081799824, 20.00000000000000000, -193.6684549073582389 ) ) ;
#1570=CIRCLE ( 'NONE', #9020, 2.000000000000000444 ) ;
#1573=DIRECTION ( 'NONE',  ( -0.000000000000000000, -1.000000000000000000, 0.000000000000000000 ) ) ;
#1579=ORIENTED_EDGE ( 'NONE', *, *, #8609, .T. ) ;
#1581=EDGE_LOOP ( 'NONE', ( #11025, #11383 ) ) ;
#1589=CARTESIAN_POINT ( 'NONE',  ( 294.1869546181097235, -19.00000000000000000, 31.92980917095290749 ) ) ;
#1594=ORIENTED_EDGE ( 'NONE', *, *, #9005, .T. ) ;
#1601=CARTESIAN_POINT ( 'NONE',  ( 185.9653539490014111, -19.00000000000000000, 225.1241593668316625 ) ) ;
#1605=CARTESIAN_POINT ( 'NONE',  ( 135.8846079354933352, -30.00000000000000000, -256.1940150085812888 ) ) ;
#1610=AXIS2_PLACEMENT_3D ( 'NONE', #2610, #1555, #11696 ) ;
#1613=EDGE_LOOP ( 'NONE', ( #1135, #1114, #5557, #3703 ) ) ;
#1615=FACE_BOUND ( 'NONE', #10482, .T. ) ;
#1619=FACE_OUTER_BOUND ( 'NONE', #958, .T. ) ;
#1621=DIRECTION ( 'NONE',  ( -0.000000000000000000, -1.000000000000000000, 0.000000000000000000 ) ) ;
#1633=ORIENTED_EDGE ( 'NONE', *, *, #8745, .F. ) ;
#1638=ORIENTED_EDGE ( 'NONE', *, *, #12741, .T. ) ;
#1639=CARTESIAN_POINT ( 'NONE',  ( -221.6213872890270977, -29.00000000000000000, 190.2057062658400923 ) ) ;
#1640=FACE_OUTER_BOUND ( 'NONE', #10969, .T. ) ;
#1641=DIRECTION ( 'NONE',  ( -0.000000000000000000, -1.000000000000000000, 0.000000000000000000 ) ) ;
#1651=EDGE_LOOP ( 'NONE', ( #9963, #7430, #3042, #2675 ) ) ;
#1652=ADVANCED_FACE ( 'NONE', ( #9945, #11211 ), #2077, .F. ) ;
#1659=DIRECTION ( 'NONE',  ( 0.6368676505102716101, 0.000000000000000000, 0.7709731485165527420 ) ) ;
#1661=DIRECTION ( 'NONE',  ( -0.4503334343941627904, -0.7071067811865381358, -0.5451603414288054283 ) ) ;
#1662=CARTESIAN_POINT ( 'NONE',  ( -290.6841825403030839, -30.00000000000000000, -27.68945685411394919 ) ) ;
#1672=ORIENTED_EDGE ( 'NONE', *, *, #4894, .F. ) ;
#1673=EDGE_LOOP ( 'NONE', ( #4388, #2858 ) ) ;
#1675=DIRECTION ( 'NONE',  ( 0.000000000000000000, 1.000000000000000000, 0.000000000000000000 ) ) ;
#1679=AXIS2_PLACEMENT_3D ( 'NONE', #1125, #8059, #931 ) ;
#1680=CIRCLE ( 'NONE', #1258, 2.500000000000025313 ) ;
#1689=AXIS2_PLACEMENT_3D ( 'NONE', #11529, #5578, #3440 ) ;
#1692=ORIENTED_EDGE ( 'NONE', *, *, #2881, .T. ) ;
#1709=CIRCLE ( 'NONE', #4673, 5.500000000000015099 ) ;
#1712=FACE_OUTER_BOUND ( 'NONE', #7058, .T. ) ;
#1719=ORIENTED_EDGE ( 'NONE', *, *, #9961, .T. ) ;
#1722=ORIENTED_EDGE ( 'NONE', *, *, #12793, .T. ) ;
#1723=EDGE_CURVE ( 'NONE', #11697, #10031, #10016, .T. ) ;
#1725=VERTEX_POINT ( 'NONE', #1951 ) ;
#1730=DIRECTION ( 'NONE',  ( -0.000000000000000000, -1.000000000000000000, 0.000000000000000000 ) ) ;
#1734=DIRECTION ( 'NONE',  ( -0.6368676505102698338, 0.000000000000000000, -0.7709731485165541853 ) ) ;
#1736=DIRECTION ( 'NONE',  ( 0.4503334343941626794, -0.7071067811865380248, 0.5451603414288055394 ) ) ;
#1745=EDGE_LOOP ( 'NONE', ( #4372, #10086 ) ) ;
#1747=FACE_BOUND ( 'NONE', #7385, .T. ) ;
#1748=ADVANCED_FACE ( 'NONE', ( #12150 ), #12548, .T. ) ;
#1751=DIRECTION ( 'NONE',  ( 0.6368676505102716101, 0.000000000000000000, 0.7709731485165527420 ) ) ;
#1754=AXIS2_PLACEMENT_3D ( 'NONE', #1307, #8638, #7507 ) ;
#1755=CARTESIAN_POINT ( 'NONE',  ( -286.5648042451072115, -19.40000000000000213, 14.34944810630078393 ) ) ;
#1758=EDGE_CURVE ( 'NONE', #169, #11069, #11704, .T. ) ;
#1761=ORIENTED_EDGE ( 'NONE', *, *, #11687, .T. ) ;
#1763=ORIENTED_EDGE ( 'NONE', *, *, #9005, .F. ) ;
#1765=CIRCLE ( 'NONE', #11335, 250.1999999999999602 ) ;
#1771=( NAMED_UNIT ( * ) SI_UNIT ( $, .STERADIAN. ) SOLID_ANGLE_UNIT ( ) );
#1772=DIRECTION ( 'NONE',  ( 0.4503334343941562956, -0.7071067811865480168, 0.5451603414287978788 ) ) ;
#1775=CIRCLE ( 'NONE', #4735, 2.000000000000000444 ) ;
#1777=VECTOR ( 'NONE', #3678, 1000.000000000000000 ) ;
#1779=ORIENTED_EDGE ( 'NONE', *, *, #1434, .F. ) ;
#1781=AXIS2_PLACEMENT_3D ( 'NONE', #3671, #5814, #5882 ) ;
#1785=AXIS2_PLACEMENT_3D ( 'NONE', #3701, #10704, #8643 ) ;
#1794=AXIS2_PLACEMENT_3D ( 'NONE', #8969, #7970, #1096 ) ;
#1795=ORIENTED_EDGE ( 'NONE', *, *, #8602, .T. ) ;
#1801=AXIS2_PLACEMENT_3D ( 'NONE', #3853, #3046, #7061 ) ;
#1803=ADVANCED_FACE ( 'NONE', ( #9351 ), #6808, .F. ) ;
#1807=AXIS2_PLACEMENT_3D ( 'NONE', #10386, #9396, #11401 ) ;
#1816=CARTESIAN_POINT ( 'NONE',  ( 192.8974817588416784, -30.00000000000000000, -159.3442861576696998 ) ) ;
#1820=CYLINDRICAL_SURFACE ( 'NONE', #1832, 250.1999999999999602 ) ;
#1827=EDGE_LOOP ( 'NONE', ( #6840, #4915 ) ) ;
#1828=EDGE_CURVE ( 'NONE', #6569, #4077, #6592, .T. ) ;
#1832=AXIS2_PLACEMENT_3D ( 'NONE', #5888, #814, #4877 ) ;
#1841=EDGE_LOOP ( 'NONE', ( #2251, #12872 ) ) ;
#1848=FACE_OUTER_BOUND ( 'NONE', #8984, .T. ) ;
#1855=EDGE_LOOP ( 'NONE', ( #6438, #8683, #1233, #4846 ) ) ;
#1858=VERTEX_POINT ( 'NONE', #6222 ) ;
#1859=CIRCLE ( 'NONE', #10578, 5.500000000000015099 ) ;
#1865=DIRECTION ( 'NONE',  ( -0.4503334343941556295, 0.7071067811865489050, -0.5451603414287969906 ) ) ;
#1866=AXIS2_PLACEMENT_3D ( 'NONE', #7709, #5710, #9769 ) ;
#1869=DIRECTION ( 'NONE',  ( 0.6368676505102696117, 0.000000000000000000, 0.7709731485165545184 ) ) ;
#1871=CARTESIAN_POINT ( 'NONE',  ( -160.3845033201291130, -9.830508068730530624, -194.1567379013694392 ) ) ;
#1875=CARTESIAN_POINT ( 'NONE',  ( -0.000000000000000000, -19.00000000000000000, 0.000000000000000000 ) ) ;
#1888=AXIS2_PLACEMENT_3D ( 'NONE', #9686, #2619, #830 ) ;
#1889=ORIENTED_EDGE ( 'NONE', *, *, #7552, .T. ) ;
#1892=ORIENTED_EDGE ( 'NONE', *, *, #10963, .T. ) ;
#1897=CARTESIAN_POINT ( 'NONE',  ( -0.000000000000000000, -29.00000000000000000, 0.000000000000000000 ) ) ;
#1900=AXIS2_PLACEMENT_3D ( 'NONE', #7905, #11788, #10776 ) ;
#1911=FACE_OUTER_BOUND ( 'NONE', #7471, .T. ) ;
#1913=LINE ( 'NONE', #4039, #11378 ) ;
#1921=VERTEX_POINT ( 'NONE', #4462 ) ;
#1923=ORIENTED_EDGE ( 'NONE', *, *, #3172, .F. ) ;
#1933=EDGE_CURVE ( 'NONE', #8227, #2601, #7478, .T. ) ;
#1935=CARTESIAN_POINT ( 'NONE',  ( 160.3845033201972115, 9.830508068689120194, 194.1567379014519190 ) ) ;
#1939=DIRECTION ( 'NONE',  ( -0.000000000000000000, -1.000000000000000000, 0.000000000000000000 ) ) ;
#1941=DIRECTION ( 'NONE',  ( 0.6368676505102716101, 0.000000000000000000, 0.7709731485165527420 ) ) ;
#1944=VECTOR ( 'NONE', #7171, 1000.000000000000000 ) ;
#1948=AXIS2_PLACEMENT_3D ( 'NONE', #6107, #6843, #5979 ) ;
#1949=VERTEX_POINT ( 'NONE', #8510 ) ;
#1951=CARTESIAN_POINT ( 'NONE',  ( 220.9845196385168435, -18.00000000000000000, -190.9766794143566528 ) ) ;
#1953=VERTEX_POINT ( 'NONE', #12799 ) ;
#1955=CARTESIAN_POINT ( 'NONE',  ( 193.6077657551222444, -30.00000000000000000, 234.3758371490322929 ) ) ;
#1961=CARTESIAN_POINT ( 'NONE',  ( 0.000000000000000000, 11.79660968244693997, 0.000000000000000000 ) ) ;
#1963=ADVANCED_FACE ( 'NONE', ( #6749 ), #4471, .F. ) ;
#1967=CIRCLE ( 'NONE', #12190, 6.500000000000000888 ) ;
#1970=VERTEX_POINT ( 'NONE', #8614 ) ;
#1973=EDGE_CURVE ( 'NONE', #2919, #1170, #11616, .T. ) ;
#1977=CARTESIAN_POINT ( 'NONE',  ( -159.3442861576697283, -21.50000000000000000, -192.8974817588416499 ) ) ;
#1981=ORIENTED_EDGE ( 'NONE', *, *, #5179, .F. ) ;
#1984=EDGE_LOOP ( 'NONE', ( #4294, #12312 ) ) ;
#1989=CIRCLE ( 'NONE', #7312, 6.500000000000005329 ) ;
#2009=CONICAL_SURFACE ( 'NONE', #9393, 250.7000000000000171, 0.7853981633974476129 ) ;
#2010=DIRECTION ( 'NONE',  ( 0.4503334343941626794, -0.7071067811865380248, 0.5451603414288055394 ) ) ;
#2013=DIRECTION ( 'NONE',  ( 0.6368676505102696117, 0.000000000000000000, 0.7709731485165545184 ) ) ;
#2017=ORIENTED_EDGE ( 'NONE', *, *, #6903, .F. ) ;
#2021=ORIENTED_EDGE ( 'NONE', *, *, #5983, .F. ) ;
#2023=DIRECTION ( 'NONE',  ( -0.000000000000000000, -1.000000000000000000, 0.000000000000000000 ) ) ;
#2026=CIRCLE ( 'NONE', #6509, 269.0000000000000000 ) ;
#2027=DIRECTION ( 'NONE',  ( -0.6368676505102707219, 0.000000000000000000, -0.7709731485165536302 ) ) ;
#2037=DIRECTION ( 'NONE',  ( 0.6368676505102700558, 0.000000000000000000, 0.7709731485165541853 ) ) ;
#2038=DIRECTION ( 'NONE',  ( 0.6368676505102716101, 0.000000000000000000, 0.7709731485165527420 ) ) ;
#2046=ORIENTED_EDGE ( 'NONE', *, *, #6198, .T. ) ;
#2050=ORIENTED_EDGE ( 'NONE', *, *, #9486, .F. ) ;
#2063=CARTESIAN_POINT ( 'NONE',  ( 153.9282213272189495, -19.40000000000000213, 245.7765299597151341 ) ) ;
#2068=LINE ( 'NONE', #3259, #10208 ) ;
#2076=VERTEX_POINT ( 'NONE', #2568 ) ;
#2077=PLANE ( 'NONE',  #8082 ) ;
#2079=VERTEX_POINT ( 'NONE', #518 ) ;
#2094=VERTEX_POINT ( 'NONE', #4310 ) ;
#2095=CARTESIAN_POINT ( 'NONE',  ( -0.000000000000000000, -30.00000000000000000, 0.000000000000000000 ) ) ;
#2099=CARTESIAN_POINT ( 'NONE',  ( -289.8128292627096130, -30.00000000000000000, 10.41748504886635907 ) ) ;
#2103=AXIS2_PLACEMENT_3D ( 'NONE', #960, #11152, #10021 ) ;
#2104=CARTESIAN_POINT ( 'NONE',  ( 153.9282213272189495, -30.00000000000000000, 245.7765299597151341 ) ) ;
#2107=FACE_OUTER_BOUND ( 'NONE', #1347, .T. ) ;
#2108=CONICAL_SURFACE ( 'NONE', #3375, 5.100000000000017408, 0.7853981633974503884 ) ;
#2110=ORIENTED_EDGE ( 'NONE', *, *, #10806, .T. ) ;
#2120=CIRCLE ( 'NONE', #2549, 5.500000000000015099 ) ;
#2121=DIRECTION ( 'NONE',  ( 0.6368676505102706109, 0.000000000000000000, 0.7709731485165535192 ) ) ;
#2123=ADVANCED_FACE ( 'NONE', ( #8519 ), #2981, .T. ) ;
#2124=DIRECTION ( 'NONE',  ( -0.000000000000000000, -1.000000000000000000, 0.000000000000000000 ) ) ;
#2134=EDGE_CURVE ( 'NONE', #11817, #3319, #10441, .T. ) ;
#2146=ORIENTED_EDGE ( 'NONE', *, *, #2336, .T. ) ;
#2151=EDGE_CURVE ( 'NONE', #8455, #10757, #639, .T. ) ;
#2155=ORIENTED_EDGE ( 'NONE', *, *, #8928, .T. ) ;
#2161=AXIS2_PLACEMENT_3D ( 'NONE', #3025, #3094, #7305 ) ;
#2168=EDGE_CURVE ( 'NONE', #11817, #6957, #8586, .T. ) ;
#2179=ORIENTED_EDGE ( 'NONE', *, *, #1023, .F. ) ;
#2199=EDGE_LOOP ( 'NONE', ( #2226, #4900, #6796, #3552 ) ) ;
#2202=AXIS2_PLACEMENT_3D ( 'NONE', #1816, #1675, #613 ) ;
#2203=EDGE_CURVE ( 'NONE', #10757, #12935, #1318, .T. ) ;
#2204=LINE ( 'NONE', #4264, #3582 ) ;
#2205=EDGE_CURVE ( 'NONE', #9116, #7165, #10575, .T. ) ;
#2216=ORIENTED_EDGE ( 'NONE', *, *, #2809, .T. ) ;
#2217=ORIENTED_EDGE ( 'NONE', *, *, #12585, .T. ) ;
#2220=DIRECTION ( 'NONE',  ( 0.6368676505102696117, 0.000000000000000000, 0.7709731485165545184 ) ) ;
#2226=ORIENTED_EDGE ( 'NONE', *, *, #7100, .F. ) ;
#2232=EDGE_LOOP ( 'NONE', ( #7992, #8033 ) ) ;
#2238=CARTESIAN_POINT ( 'NONE',  ( -286.5648042451072115, -30.00000000000000000, 14.34944810630078393 ) ) ;
#2240=CARTESIAN_POINT ( 'NONE',  ( -24.18668477630637526, -19.00000000000000000, 294.9245348571438967 ) ) ;
#2241=DIRECTION ( 'NONE',  ( 0.6368676505102708330, 0.000000000000000000, 0.7709731485165535192 ) ) ;
#2248=DIRECTION ( 'NONE',  ( 0.000000000000000000, 1.000000000000000000, 0.000000000000000000 ) ) ;
#2251=ORIENTED_EDGE ( 'NONE', *, *, #1303, .T. ) ;
#2257=( NAMED_UNIT ( * ) SI_UNIT ( $, .STERADIAN. ) SOLID_ANGLE_UNIT ( ) );
#2270=CARTESIAN_POINT ( 'NONE',  ( 153.9282213272189495, -19.40000000000000213, 245.7765299597151341 ) ) ;
#2275=VERTEX_POINT ( 'NONE', #3364 ) ;
#2276=EDGE_LOOP ( 'NONE', ( #679, #4432, #859, #9482 ) ) ;
#2277=DIRECTION ( 'NONE',  ( 0.4503334343941562401, 0.7071067811865480168, 0.5451603414287978788 ) ) ;
#2282=CARTESIAN_POINT ( 'NONE',  ( -0.000000000000000000, -18.00000000000000000, 0.000000000000000000 ) ) ;
#2288=DIRECTION ( 'NONE',  ( 0.000000000000000000, 1.000000000000000000, 0.000000000000000000 ) ) ;
#2294=ADVANCED_FACE ( 'NONE', ( #11521 ), #5514, .F. ) ;
#2299=DIRECTION ( 'NONE',  ( 0.6368676505102700558, 0.000000000000000000, 0.7709731485165541853 ) ) ;
#2306=DIRECTION ( 'NONE',  ( -0.4503334343941691187, -0.7071067811865280328, -0.5451603414288131999 ) ) ;
#2311=DIRECTION ( 'NONE',  ( 0.6368676505102700558, 0.000000000000000000, 0.7709731485165541853 ) ) ;
#2315=EDGE_CURVE ( 'NONE', #3553, #5907, #7481, .T. ) ;
#2317=VECTOR ( 'NONE', #6829, 1000.000000000000000 ) ;
#2322=SHAPE_DEFINITION_REPRESENTATION ( #10544, #11596 ) ;
#2329=ORIENTED_EDGE ( 'NONE', *, *, #1758, .T. ) ;
#2331=CARTESIAN_POINT ( 'NONE',  ( 190.1049936773181628, -18.00000000000000000, 230.1354848321892632 ) ) ;
#2335=CIRCLE ( 'NONE', #6388, 251.8333333333380608 ) ;
#2336=EDGE_CURVE ( 'NONE', #3553, #900, #3508, .T. ) ;
#2338=VECTOR ( 'NONE', #251, 1000.000000000000000 ) ;
#2339=CARTESIAN_POINT ( 'NONE',  ( 189.4681260268079086, -29.00000000000000000, 229.3645116836727027 ) ) ;
#2341=DIRECTION ( 'NONE',  ( 0.6368676505102689456, 0.000000000000000000, 0.7709731485165549625 ) ) ;
#2347=ORIENTED_EDGE ( 'NONE', *, *, #4320, .T. ) ;
#2351=FACE_BOUND ( 'NONE', #5773, .T. ) ;
#2352=AXIS2_PLACEMENT_3D ( 'NONE', #1384, #10514, #9510 ) ;
#2354=DIRECTION ( 'NONE',  ( -0.000000000000000000, -1.000000000000000000, 0.000000000000000000 ) ) ;
#2361=VERTEX_POINT ( 'NONE', #454 ) ;
#2365=CARTESIAN_POINT ( 'NONE',  ( -165.7021400752470015, 1.848645179581459796, -200.5941117395221056 ) ) ;
#2371=DIRECTION ( 'NONE',  ( 0.6368676505102716101, 0.000000000000000000, 0.7709731485165527420 ) ) ;
#2372=FACE_OUTER_BOUND ( 'NONE', #6366, .T. ) ;
#2374=ORIENTED_EDGE ( 'NONE', *, *, #9725, .T. ) ;
#2376=CARTESIAN_POINT ( 'NONE',  ( 182.4625818711949137, -30.00000000000000000, 220.8838070499906223 ) ) ;
#2377=ORIENTED_EDGE ( 'NONE', *, *, #2854, .T. ) ;
#2378=CARTESIAN_POINT ( 'NONE',  ( -185.9653539489998195, -18.00000000000000000, -225.1241593668329699 ) ) ;
#2385=LINE ( 'NONE', #1325, #10371 ) ;
#2386=CONICAL_SURFACE ( 'NONE', #894, 6.500000000000005329, 0.7853981633974518317 ) ;
#2392=DIRECTION ( 'NONE',  ( -0.4503334343941556295, 0.7071067811865489050, -0.5451603414287969906 ) ) ;
#2394=VECTOR ( 'NONE', #10876, 1000.000000000000114 ) ;
#2403=AXIS2_PLACEMENT_3D ( 'NONE', #7014, #10076, #11206 ) ;
#2408=CARTESIAN_POINT ( 'NONE',  ( 31.19222893192144852, -29.00000000000000000, -286.4438302234616458 ) ) ;
#2410=EDGE_LOOP ( 'NONE', ( #5759, #9455, #2377, #3932 ) ) ;
#2413=AXIS2_PLACEMENT_3D ( 'NONE', #8506, #3492, #5495 ) ;
#2421=DIRECTION ( 'NONE',  ( 0.6368676505102695007, 0.000000000000000000, 0.7709731485165545184 ) ) ;
#2426=FACE_OUTER_BOUND ( 'NONE', #1855, .T. ) ;
#2431=DIRECTION ( 'NONE',  ( -0.4503334343941563511, -0.7071067811865480168, -0.5451603414287977678 ) ) ;
#2435=CARTESIAN_POINT ( 'NONE',  ( -225.1241593668336236, -18.00000000000000000, 185.9653539489990521 ) ) ;
#2446=DIRECTION ( 'NONE',  ( 0.000000000000000000, -1.000000000000000000, 0.000000000000000000 ) ) ;
#2449=VECTOR ( 'NONE', #3995, 1000.000000000000000 ) ;
#2462=CARTESIAN_POINT ( 'NONE',  ( 27.68945685411497593, -30.00000000000000000, -290.6841825403026291 ) ) ;
#2472=DIRECTION ( 'NONE',  ( 0.6368676505102696117, 0.000000000000000000, 0.7709731485165545184 ) ) ;
#2473=ORIENTED_EDGE ( 'NONE', *, *, #2854, .F. ) ;
#2483=DIRECTION ( 'NONE',  ( 0.6368676505102707219, 0.000000000000000000, 0.7709731485165535192 ) ) ;
#2485=ORIENTED_EDGE ( 'NONE', *, *, #2315, .F. ) ;
#2487=EDGE_CURVE ( 'NONE', #9382, #4412, #7903, .T. ) ;
#2489=AXIS2_PLACEMENT_3D ( 'NONE', #6494, #291, #9536 ) ;
#2490=DIRECTION ( 'NONE',  ( 0.6368676505102696117, 0.000000000000000000, 0.7709731485165545184 ) ) ;
#2493=CARTESIAN_POINT ( 'NONE',  ( -190.1049936773165996, -30.00000000000000000, -230.1354848321905706 ) ) ;
#2499=EDGE_LOOP ( 'NONE', ( #4914, #8787, #7367, #4008 ) ) ;
#2519=VECTOR ( 'NONE', #5676, 1000.000000000000000 ) ;
#2522=CARTESIAN_POINT ( 'NONE',  ( -0.000000000000000000, -30.00000000000000000, 0.000000000000000000 ) ) ;
#2526=DIRECTION ( 'NONE',  ( -0.000000000000000000, -1.000000000000000000, 0.000000000000000000 ) ) ;
#2531=CONICAL_SURFACE ( 'NONE', #9548, 305.0000000000000000, 0.7853981633974758125 ) ;
#2539=VERTEX_POINT ( 'NONE', #11975 ) ;
#2543=FACE_BOUND ( 'NONE', #10166, .T. ) ;
#2549=AXIS2_PLACEMENT_3D ( 'NONE', #1601, #598, #3656 ) ;
#2552=DIRECTION ( 'NONE',  ( 0.000000000000000000, 1.000000000000000000, 0.000000000000000000 ) ) ;
#2554=EDGE_LOOP ( 'NONE', ( #4704, #6063, #1692, #10918 ) ) ;
#2556=EDGE_CURVE ( 'NONE', #10957, #327, #9818, .T. ) ;
#2558=CARTESIAN_POINT ( 'NONE',  ( -225.1241593668336236, -30.00000000000000000, 185.9653539489990521 ) ) ;
#2568=CARTESIAN_POINT ( 'NONE',  ( -171.3173979872628649, 20.00000000000000000, -207.3917769509529023 ) ) ;
#2573=CARTESIAN_POINT ( 'NONE',  ( 159.3442861576696998, -29.00000000000000000, 192.8974817588416784 ) ) ;
#2574=DIRECTION ( 'NONE',  ( 0.4503334343941562956, -0.7071067811865480168, 0.5451603414287978788 ) ) ;
#2576=DIRECTION ( 'NONE',  ( -0.6368676505102707219, 0.000000000000000000, -0.7709731485165536302 ) ) ;
#2577=AXIS2_PLACEMENT_3D ( 'NONE', #4768, #11787, #6782 ) ;
#2579=DIRECTION ( 'NONE',  ( -0.6368676505102708330, 0.000000000000000000, -0.7709731485165536302 ) ) ;
#2589=CARTESIAN_POINT ( 'NONE',  ( -290.6841825403030839, -29.00000000000000000, -27.68945685411394919 ) ) ;
#2591=CARTESIAN_POINT ( 'NONE',  ( -27.68945685411286561, -19.00000000000000000, 290.6841825403027997 ) ) ;
#2593=DIRECTION ( 'NONE',  ( 0.6368676505102707219, 0.000000000000000000, 0.7709731485165535192 ) ) ;
#2595=AXIS2_PLACEMENT_3D ( 'NONE', #2779, #11221, #7231 ) ;
#2601=VERTEX_POINT ( 'NONE', #1639 ) ;
#2602=EDGE_CURVE ( 'NONE', #11697, #2539, #3635, .T. ) ;
#2606=FACE_OUTER_BOUND ( 'NONE', #9434, .T. ) ;
#2610=CARTESIAN_POINT ( 'NONE',  ( 0.000000000000000000, 3.327561323230709966, 0.000000000000000000 ) ) ;
#2615=VECTOR ( 'NONE', #10566, 1000.000000000000000 ) ;
#2618=VERTEX_POINT ( 'NONE', #9766 ) ;
#2619=DIRECTION ( 'NONE',  ( 0.000000000000000000, 1.000000000000000000, 0.000000000000000000 ) ) ;
#2622=DIRECTION ( 'NONE',  ( -0.000000000000000000, -1.000000000000000000, 0.000000000000000000 ) ) ;
#2629=ORIENTED_EDGE ( 'NONE', *, *, #10487, .F. ) ;
#2634=DIRECTION ( 'NONE',  ( 0.6368676505102709440, 0.000000000000000000, 0.7709731485165532971 ) ) ;
#2635=CARTESIAN_POINT ( 'NONE',  ( -159.3442861576697283, -25.50000000000000000, -192.8974817588417068 ) ) ;
#2638=EDGE_CURVE ( 'NONE', #6987, #5762, #8775, .T. ) ;
#2640=VERTEX_POINT ( 'NONE', #7773 ) ;
#2649=CARTESIAN_POINT ( 'NONE',  ( -165.3358371128620661, -2.772967769358684720, -200.1506762031204971 ) ) ;
#2650=LINE ( 'NONE', #11999, #2940 ) ;
#2660=AXIS2_PLACEMENT_3D ( 'NONE', #10499, #8438, #9435 ) ;
#2669=DIRECTION ( 'NONE',  ( -0.6368676505102707219, 0.000000000000000000, -0.7709731485165535192 ) ) ;
#2671=ADVANCED_FACE ( 'NONE', ( #8040 ), #4968, .F. ) ;
#2673=CARTESIAN_POINT ( 'NONE',  ( -159.3442861576697283, -21.50000000000000000, -192.8974817588416499 ) ) ;
#2675=ORIENTED_EDGE ( 'NONE', *, *, #2168, .F. ) ;
#2681=CARTESIAN_POINT ( 'NONE',  ( 135.8846079354933352, -28.60000000000000142, -256.1940150085812888 ) ) ;
#2683=LINE ( 'NONE', #2884, #9631 ) ;
#2690=VERTEX_POINT ( 'NONE', #5094 ) ;
#2691=EDGE_CURVE ( 'NONE', #9851, #12208, #11743, .T. ) ;
#2694=CARTESIAN_POINT ( 'NONE',  ( 0.000000000000000000, 19.00000000000000000, 0.000000000000000000 ) ) ;
#2698=CARTESIAN_POINT ( 'NONE',  ( -0.000000000000000000, -2.772967769358684720, 0.000000000000000000 ) ) ;
#2700=ORIENTED_EDGE ( 'NONE', *, *, #161, .F. ) ;
#2701=CARTESIAN_POINT ( 'NONE',  ( -286.5445428119863891, -18.00000000000000000, -22.67813138875635204 ) ) ;
#2708=ADVANCED_FACE ( 'NONE', ( #11168 ), #9239, .F. ) ;
#2710=CARTESIAN_POINT ( 'NONE',  ( -159.3442861576696998, -11.79660968244695951, -192.8974817588416784 ) ) ;
#2712=EDGE_CURVE ( 'NONE', #3319, #7354, #6106, .T. ) ;
#2748=FACE_OUTER_BOUND ( 'NONE', #5287, .T. ) ;
#2751=VERTEX_POINT ( 'NONE', #5233 ) ;
#2754=EDGE_CURVE ( 'NONE', #11433, #779, #908, .T. ) ;
#2766=ORIENTED_EDGE ( 'NONE', *, *, #8533, .F. ) ;
#2771=ORIENTED_EDGE ( 'NONE', *, *, #8334, .F. ) ;
#2773=EDGE_LOOP ( 'NONE', ( #7756, #11313, #9549, #6631 ) ) ;
#2776=CARTESIAN_POINT ( 'NONE',  ( -189.4681260268063170, -29.00000000000000000, -229.3645116836740101 ) ) ;
#2777=DIRECTION ( 'NONE',  ( 0.4503334343941555740, 0.7071067811865490160, 0.5451603414287971017 ) ) ;
#2779=CARTESIAN_POINT ( 'NONE',  ( 27.68945685411497593, -30.00000000000000000, -290.6841825403026291 ) ) ;
#2780=CARTESIAN_POINT ( 'NONE',  ( -166.5596220099214690, 3.327561323230709966, -201.6321540179175713 ) ) ;
#2785=AXIS2_PLACEMENT_3D ( 'NONE', #10039, #7242, #975 ) ;
#2790=ORIENTED_EDGE ( 'NONE', *, *, #1933, .T. ) ;
#2792=AXIS2_PLACEMENT_3D ( 'NONE', #12863, #8610, #11810 ) ;
#2801=AXIS2_PLACEMENT_3D ( 'NONE', #1359, #2354, #8431 ) ;
#2805=CIRCLE ( 'NONE', #8785, 6.500000000000005329 ) ;
#2809=EDGE_CURVE ( 'NONE', #8685, #10853, #5133, .T. ) ;
#2815=LINE ( 'NONE', #3694, #9660 ) ;
#2817=DIRECTION ( 'NONE',  ( -0.4503334343941563511, -0.7071067811865480168, -0.5451603414287977678 ) ) ;
#2821=AXIS2_PLACEMENT_3D ( 'NONE', #6321, #10238, #9312 ) ;
#2830=CONICAL_SURFACE ( 'NONE', #1794, 5.500000000000015099, 0.7853981633974461696 ) ;
#2837=ADVANCED_FACE ( 'NONE', ( #11103 ), #10246, .F. ) ;
#2838=VERTEX_POINT ( 'NONE', #113 ) ;
#2844=CARTESIAN_POINT ( 'NONE',  ( 0.000000000000000000, 3.327561323230709966, 0.000000000000000000 ) ) ;
#2845=CARTESIAN_POINT ( 'NONE',  ( -0.000000000000000000, -29.00000000000000000, 0.000000000000000000 ) ) ;
#2846=AXIS2_PLACEMENT_3D ( 'NONE', #4503, #2446, #8589 ) ;
#2851=AXIS2_PLACEMENT_3D ( 'NONE', #5939, #12268, #1869 ) ;
#2853=DIRECTION ( 'NONE',  ( 0.4503334343941555740, 0.7071067811865490160, 0.5451603414287971017 ) ) ;
#2854=EDGE_CURVE ( 'NONE', #4077, #6569, #8756, .T. ) ;
#2858=ORIENTED_EDGE ( 'NONE', *, *, #9265, .F. ) ;
#2859=AXIS2_PLACEMENT_3D ( 'NONE', #12266, #11259, #2121 ) ;
#2863=EDGE_CURVE ( 'NONE', #7702, #9318, #10461, .T. ) ;
#2865=CARTESIAN_POINT ( 'NONE',  ( 181.8257142206846311, -30.00000000000000000, 220.1128339014740618 ) ) ;
#2871=DIRECTION ( 'NONE',  ( -0.7709731485165535192, 0.000000000000000000, 0.6368676505102708330 ) ) ;
#2872=DIRECTION ( 'NONE',  ( -0.000000000000000000, -1.000000000000000000, 0.000000000000000000 ) ) ;
#2873=EDGE_LOOP ( 'NONE', ( #5833, #8453, #10259, #95 ) ) ;
#2877=EDGE_LOOP ( 'NONE', ( #7953, #1892, #6337, #567 ) ) ;
#2879=AXIS2_PLACEMENT_3D ( 'NONE', #2931, #9018, #12281 ) ;
#2880=CARTESIAN_POINT ( 'NONE',  ( 185.9653539490014111, -18.00000000000000000, 225.1241593668316625 ) ) ;
#2881=EDGE_CURVE ( 'NONE', #11832, #3272, #12213, .T. ) ;
#2884=CARTESIAN_POINT ( 'NONE',  ( 149.7885815989021694, -30.00000000000000000, 240.7652044943575333 ) ) ;
#2899=UNCERTAINTY_MEASURE_WITH_UNIT (LENGTH_MEASURE( 1.000000000000000082E-05 ), #10895, 'distance_accuracy_value', 'NONE');
#2901=DIRECTION ( 'NONE',  ( 0.4503334343941441387, 0.7071067811865670016, 0.5451603414287832239 ) ) ;
#2908=FACE_OUTER_BOUND ( 'NONE', #284, .T. ) ;
#2918=CARTESIAN_POINT ( 'NONE',  ( 135.8846079354933352, -18.00000000000000000, -256.1940150085812888 ) ) ;
#2919=VERTEX_POINT ( 'NONE', #438 ) ;
#2923=EDGE_CURVE ( 'NONE', #11199, #354, #5298, .T. ) ;
#2924=EDGE_CURVE ( 'NONE', #3236, #11029, #372, .T. ) ;
#2925=CARTESIAN_POINT ( 'NONE',  ( 153.9282213272189495, -28.60000000000000142, 245.7765299597151341 ) ) ;
#2929=DIRECTION ( 'NONE',  ( -0.4503334343941595708, -0.7071067811865430208, -0.5451603414288016536 ) ) ;
#2931=CARTESIAN_POINT ( 'NONE',  ( 27.68945685411497593, -29.00000000000000000, -290.6841825403026291 ) ) ;
#2937=EDGE_LOOP ( 'NONE', ( #11224, #5310, #8901, #79 ) ) ;
#2938=AXIS2_PLACEMENT_3D ( 'NONE', #893, #11408, #12157 ) ;
#2939=EDGE_LOOP ( 'NONE', ( #10376, #8742, #1889, #856 ) ) ;
#2940=VECTOR ( 'NONE', #666, 999.9999999999998863 ) ;
#2941=CARTESIAN_POINT ( 'NONE',  ( 0.000000000000000000, 0.000000000000000000, 0.000000000000000000 ) ) ;
#2942=LINE ( 'NONE', #11153, #11685 ) ;
#2944=VECTOR ( 'NONE', #8501, 999.9999999999998863 ) ;
#2945=CIRCLE ( 'NONE', #12967, 5.500000000000015099 ) ;
#2947=CONICAL_SURFACE ( 'NONE', #10949, 270.0000000000000000, 0.7853981633974476129 ) ;
#2952=CONICAL_SURFACE ( 'NONE', #1265, 250.7000000000000171, 0.7853981633974476129 ) ;
#2956=ORIENTED_EDGE ( 'NONE', *, *, #607, .F. ) ;
#2960=AXIS2_PLACEMENT_3D ( 'NONE', #9306, #6443, #9374 ) ;
#2961=CARTESIAN_POINT ( 'NONE',  ( 159.3442861576696998, 0.000000000000000000, 192.8974817588416784 ) ) ;
#2962=FACE_OUTER_BOUND ( 'NONE', #3431, .T. ) ;
#2966=DIRECTION ( 'NONE',  ( -0.000000000000000000, -1.000000000000000000, 0.000000000000000000 ) ) ;
#2972=VERTEX_POINT ( 'NONE', #1372 ) ;
#2973=ADVANCED_FACE ( 'NONE', ( #7434 ), #10630, .T. ) ;
#2979=DIRECTION ( 'NONE',  ( -0.6368676505102707219, 0.000000000000000000, -0.7709731485165535192 ) ) ;
#2981=TOROIDAL_SURFACE ( 'NONE', #9379, 261.5294117647060261, 2.000000000000000000 ) ;
#2991=EDGE_CURVE ( 'NONE', #4661, #4062, #8892, .T. ) ;
#2997=CARTESIAN_POINT ( 'NONE',  ( -182.4625818711933221, -30.00000000000000000, -220.8838070499919013 ) ) ;
#3001=AXIS2_PLACEMENT_3D ( 'NONE', #4618, #4425, #10570 ) ;
#3003=ORIENTED_EDGE ( 'NONE', *, *, #6858, .F. ) ;
#3005=EDGE_CURVE ( 'NONE', #10483, #11299, #4486, .T. ) ;
#3009=CARTESIAN_POINT ( 'NONE',  ( 0.000000000000000000, 1.848645179581460019, 0.000000000000000000 ) ) ;
#3010=DIRECTION ( 'NONE',  ( 0.6368676505102707219, 0.000000000000000000, 0.7709731485165536302 ) ) ;
#3018=AXIS2_PLACEMENT_3D ( 'NONE', #10669, #10602, #7410 ) ;
#3023=AXIS2_PLACEMENT_3D ( 'NONE', #9428, #6497, #6361 ) ;
#3025=CARTESIAN_POINT ( 'NONE',  ( 290.6841825403032544, -30.00000000000000000, 27.68945685411186730 ) ) ;
#3028=EDGE_CURVE ( 'NONE', #8752, #8227, #11789, .T. ) ;
#3035=ORIENTED_EDGE ( 'NONE', *, *, #4231, .T. ) ;
#3038=VERTEX_POINT ( 'NONE', #2365 ) ;
#3041=DIRECTION ( 'NONE',  ( -0.7709731485165536302, 0.000000000000000000, 0.6368676505102706109 ) ) ;
#3042=ORIENTED_EDGE ( 'NONE', *, *, #10099, .T. ) ;
#3044=AXIS2_PLACEMENT_3D ( 'NONE', #7699, #8516, #1506 ) ;
#3046=DIRECTION ( 'NONE',  ( -0.000000000000000000, -1.000000000000000000, 0.000000000000000000 ) ) ;
#3049=EDGE_CURVE ( 'NONE', #4180, #2640, #5693, .T. ) ;
#3051=CARTESIAN_POINT ( 'NONE',  ( -24.18668477630638947, -29.00000000000000000, 294.9245348571438399 ) ) ;
#3053=CARTESIAN_POINT ( 'NONE',  ( 225.1241593668336236, -30.00000000000000000, -185.9653539489990521 ) ) ;
#3054=CONICAL_SURFACE ( 'NONE', #5189, 6.500000000000005329, 0.7853981633974518317 ) ;
#3062=DIRECTION ( 'NONE',  ( 0.4503334343941626794, -0.7071067811865380248, 0.5451603414288055394 ) ) ;
#3066=AXIS2_PLACEMENT_3D ( 'NONE', #2844, #4851, #10991 ) ;
#3072=ORIENTED_EDGE ( 'NONE', *, *, #10308, .T. ) ;
#3074=VECTOR ( 'NONE', #656, 1000.000000000000000 ) ;
#3082=VECTOR ( 'NONE', #8207, 1000.000000000000000 ) ;
#3087=ORIENTED_EDGE ( 'NONE', *, *, #92, .T. ) ;
#3094=DIRECTION ( 'NONE',  ( -0.000000000000000000, -1.000000000000000000, 0.000000000000000000 ) ) ;
#3099=DIRECTION ( 'NONE',  ( 0.6368676505102716101, 0.000000000000000000, 0.7709731485165527420 ) ) ;
#3100=CARTESIAN_POINT ( 'NONE',  ( -0.000000000000000000, -19.00000000000000000, 0.000000000000000000 ) ) ;
#3112=DIRECTION ( 'NONE',  ( -0.000000000000000000, -1.000000000000000000, 0.000000000000000000 ) ) ;
#3119=CARTESIAN_POINT ( 'NONE',  ( -294.1869546181095529, -29.00000000000000000, -31.92980917095497517 ) ) ;
#3120=ORIENTED_EDGE ( 'NONE', *, *, #1156, .F. ) ;
#3125=CARTESIAN_POINT ( 'NONE',  ( 171.9542656377731191, 19.00000000000000000, 208.1627500994694628 ) ) ;
#3127=DIRECTION ( 'NONE',  ( -0.7709731485165534082, 0.000000000000000000, 0.6368676505102708330 ) ) ;
#3134=CARTESIAN_POINT ( 'NONE',  ( -221.6213872890270977, -30.00000000000000000, 190.2057062658400923 ) ) ;
#3136=FACE_OUTER_BOUND ( 'NONE', #11638, .T. ) ;
#3139=DIRECTION ( 'NONE',  ( 0.6368676505102707219, 0.000000000000000000, 0.7709731485165535192 ) ) ;
#3157=DIRECTION ( 'NONE',  ( -0.000000000000000000, -1.000000000000000000, 0.000000000000000000 ) ) ;
#3159=DIRECTION ( 'NONE',  ( -0.000000000000000000, -1.000000000000000000, 0.000000000000000000 ) ) ;
#3160=DIRECTION ( 'NONE',  ( -0.4503334343941563511, -0.7071067811865480168, -0.5451603414287977678 ) ) ;
#3161=AXIS2_PLACEMENT_3D ( 'NONE', #9925, #6865, #11927 ) ;
#3164=CIRCLE ( 'NONE', #6797, 6.500000000000000888 ) ;
#3172=EDGE_CURVE ( 'NONE', #10034, #354, #1989, .T. ) ;
#3173=VECTOR ( 'NONE', #12841, 1000.000000000000000 ) ;
#3178=DIRECTION ( 'NONE',  ( -0.000000000000000000, -1.000000000000000000, 0.000000000000000000 ) ) ;
#3187=ORIENTED_EDGE ( 'NONE', *, *, #2923, .T. ) ;
#3198=CARTESIAN_POINT ( 'NONE',  ( 166.5596220099214406, 3.327561323230709966, 201.6321540179175997 ) ) ;
#3203=CARTESIAN_POINT ( 'NONE',  ( -225.1241593668336236, -19.00000000000000000, 185.9653539489990521 ) ) ;
#3207=ORIENTED_EDGE ( 'NONE', *, *, #6795, .F. ) ;
#3211=CONICAL_SURFACE ( 'NONE', #2577, 5.100000000000003197, 0.7853981633974461696 ) ;
#3227=LINE ( 'NONE', #12631, #11052 ) ;
#3236=VERTEX_POINT ( 'NONE', #9954 ) ;
#3237=VECTOR ( 'NONE', #9824, 1000.000000000000114 ) ;
#3248=EDGE_CURVE ( 'NONE', #2094, #6789, #3790, .T. ) ;
#3259=CARTESIAN_POINT ( 'NONE',  ( 189.4681260268079086, -30.00000000000000000, 229.3645116836727311 ) ) ;
#3260=DIRECTION ( 'NONE',  ( 0.4503334343941562956, -0.7071067811865480168, 0.5451603414287978788 ) ) ;
#3263=CIRCLE ( 'NONE', #3698, 259.6078431372534396 ) ;
#3264=CARTESIAN_POINT ( 'NONE',  ( 153.9282213272189495, -30.00000000000000000, 245.7765299597151341 ) ) ;
#3266=DIRECTION ( 'NONE',  ( -0.000000000000000000, -1.000000000000000000, 0.000000000000000000 ) ) ;
#3272=VERTEX_POINT ( 'NONE', #633 ) ;
#3273=EDGE_CURVE ( 'NONE', #6957, #6789, #8697, .T. ) ;
#3274=CARTESIAN_POINT ( 'NONE',  ( -293.0608542803120145, -19.40000000000000213, 6.485521991431935973 ) ) ;
#3278=CARTESIAN_POINT ( 'NONE',  ( -220.9845196385168435, -18.00000000000000000, 190.9766794143566528 ) ) ;
#3279=CIRCLE ( 'NONE', #11819, 6.500000000000005329 ) ;
#3284=ORIENTED_EDGE ( 'NONE', *, *, #1524, .F. ) ;
#3286=EDGE_CURVE ( 'NONE', #2618, #1953, #2204, .T. ) ;
#3287=EDGE_CURVE ( 'NONE', #11992, #823, #5718, .T. ) ;
#3288=STYLED_ITEM ( 'NONE', ( #4991 ), #5935 ) ;
#3292=FACE_OUTER_BOUND ( 'NONE', #12831, .T. ) ;
#3300=VECTOR ( 'NONE', #461, 1000.000000000000000 ) ;
#3307=ORIENTED_EDGE ( 'NONE', *, *, #12888, .T. ) ;
#3312=DIRECTION ( 'NONE',  ( 0.000000000000000000, 1.000000000000000000, 0.000000000000000000 ) ) ;
#3319=VERTEX_POINT ( 'NONE', #3955 ) ;
#3323=DIRECTION ( 'NONE',  ( 0.6368676505102716101, 0.000000000000000000, 0.7709731485165527420 ) ) ;
#3324=DIRECTION ( 'NONE',  ( 0.6368676505102716101, 0.000000000000000000, 0.7709731485165527420 ) ) ;
#3334=ORIENTED_EDGE ( 'NONE', *, *, #895, .F. ) ;
#3337=CARTESIAN_POINT ( 'NONE',  ( -190.1049936773165996, -30.00000000000000000, -230.1354848321905706 ) ) ;
#3339=DIRECTION ( 'NONE',  ( 0.6368676505102716101, 0.000000000000000000, 0.7709731485165527420 ) ) ;
#3343=ORIENTED_EDGE ( 'NONE', *, *, #8129, .F. ) ;
#3347=ORIENTED_EDGE ( 'NONE', *, *, #6793, .F. ) ;
#3348=ORIENTED_EDGE ( 'NONE', *, *, #8123, .T. ) ;
#3350=DIRECTION ( 'NONE',  ( -0.6368676505102707219, 0.000000000000000000, -0.7709731485165535192 ) ) ;
#3359=ADVANCED_FACE ( 'NONE', ( #4309 ), #10609, .F. ) ;
#3362=ORIENTED_EDGE ( 'NONE', *, *, #11157, .T. ) ;
#3363=DIRECTION ( 'NONE',  ( 0.000000000000000000, 1.000000000000000000, 0.000000000000000000 ) ) ;
#3364=CARTESIAN_POINT ( 'NONE',  ( -285.6731895343928613, -18.00000000000000000, 15.42881051422396332 ) ) ;
#3366=ORIENTED_EDGE ( 'NONE', *, *, #3546, .F. ) ;
#3375=AXIS2_PLACEMENT_3D ( 'NONE', #1203, #1133, #5192 ) ;
#3383=DIRECTION ( 'NONE',  ( -0.6368676505102706109, 0.000000000000000000, -0.7709731485165535192 ) ) ;
#3387=CARTESIAN_POINT ( 'NONE',  ( -164.6302876569050113, -3.165711975795909891E-14, -199.2965588915290596 ) ) ;
#3388=DIRECTION ( 'NONE',  ( 0.6368676505102689456, 0.000000000000000000, 0.7709731485165549625 ) ) ;
#3389=AXIS2_PLACEMENT_3D ( 'NONE', #4234, #3422, #9557 ) ;
#3390=FACE_OUTER_BOUND ( 'NONE', #12955, .T. ) ;
#3403=FACE_BOUND ( 'NONE', #4674, .T. ) ;
#3409=DIRECTION ( 'NONE',  ( -0.000000000000000000, -1.000000000000000000, 0.000000000000000000 ) ) ;
#3410=ADVANCED_FACE ( 'NONE', ( #128 ), #8281, .F. ) ;
#3414=EDGE_LOOP ( 'NONE', ( #2629, #3343, #3814, #1579 ) ) ;
#3418=DIRECTION ( 'NONE',  ( 0.6368676505102707219, 0.000000000000000000, 0.7709731485165535192 ) ) ;
#3419=CIRCLE ( 'NONE', #10036, 6.500000000000026645 ) ;
#3422=DIRECTION ( 'NONE',  ( 0.000000000000000000, 1.000000000000000000, 0.000000000000000000 ) ) ;
#3431=EDGE_LOOP ( 'NONE', ( #7054, #12049, #3486, #5717 ) ) ;
#3440=DIRECTION ( 'NONE',  ( 0.6368676505102707219, 0.000000000000000000, 0.7709731485165535192 ) ) ;
#3443=CARTESIAN_POINT ( 'NONE',  ( 290.6841825403032544, -29.00000000000000000, 27.68945685411186730 ) ) ;
#3449=CARTESIAN_POINT ( 'NONE',  ( 27.68945685411497593, -18.00000000000000000, -290.6841825403026291 ) ) ;
#3450=ORIENTED_EDGE ( 'NONE', *, *, #5173, .F. ) ;
#3451=CIRCLE ( 'NONE', #3023, 6.500000000000000888 ) ;
#3460=EDGE_CURVE ( 'NONE', #8072, #5762, #12105, .T. ) ;
#3464=DIRECTION ( 'NONE',  ( -0.6368676505102708330, 0.000000000000000000, -0.7709731485165536302 ) ) ;
#3470=AXIS2_PLACEMENT_3D ( 'NONE', #9875, #6690, #9672 ) ;
#3475=FACE_BOUND ( 'NONE', #5400, .T. ) ;
#3476=AXIS2_PLACEMENT_3D ( 'NONE', #710, #7895, #3962 ) ;
#3477=AXIS2_PLACEMENT_3D ( 'NONE', #7594, #4586, #6604 ) ;
#3482=FACE_OUTER_BOUND ( 'NONE', #7238, .T. ) ;
#3485=AXIS2_PLACEMENT_3D ( 'NONE', #11967, #9830, #7826 ) ;
#3486=ORIENTED_EDGE ( 'NONE', *, *, #9265, .T. ) ;
#3489=EDGE_LOOP ( 'NONE', ( #2021, #11570, #4289, #4228 ) ) ;
#3490=CIRCLE ( 'NONE', #10527, 5.499999999999986677 ) ;
#3491=EDGE_CURVE ( 'NONE', #1921, #941, #12319, .T. ) ;
#3492=DIRECTION ( 'NONE',  ( -0.000000000000000000, -1.000000000000000000, 0.000000000000000000 ) ) ;
#3493=DIRECTION ( 'NONE',  ( -0.000000000000000000, -1.000000000000000000, 0.000000000000000000 ) ) ;
#3496=VECTOR ( 'NONE', #2853, 1000.000000000000000 ) ;
#3498=CARTESIAN_POINT ( 'NONE',  ( -285.6731895343928613, -30.00000000000000000, 15.42881051422395622 ) ) ;
#3505=AXIS2_PLACEMENT_3D ( 'NONE', #1875, #13007, #3869 ) ;
#3507=ADVANCED_FACE ( 'NONE', ( #1119 ), #9509, .F. ) ;
#3508=LINE ( 'NONE', #5450, #4458 ) ;
#3509=DIRECTION ( 'NONE',  ( -0.000000000000000000, -1.000000000000000000, 0.000000000000000000 ) ) ;
#3513=CARTESIAN_POINT ( 'NONE',  ( -225.1241593668336236, -29.00000000000000000, 185.9653539489990521 ) ) ;
#3515=CONICAL_SURFACE ( 'NONE', #12040, 304.0000000000000000, 0.7853981633974207455 ) ;
#3517=DIRECTION ( 'NONE',  ( -0.000000000000000000, -1.000000000000000000, 0.000000000000000000 ) ) ;
#3529=CARTESIAN_POINT ( 'NONE',  ( -185.9653539489998195, -30.00000000000000000, -225.1241593668329699 ) ) ;
#3537=EDGE_LOOP ( 'NONE', ( #7971, #989, #8926, #6474 ) ) ;
#3538=DIRECTION ( 'NONE',  ( 0.000000000000000000, 1.000000000000000000, 0.000000000000000000 ) ) ;
#3546=EDGE_CURVE ( 'NONE', #6987, #10768, #9752, .T. ) ;
#3550=CIRCLE ( 'NONE', #2489, 6.500000000000005329 ) ;
#3551=DIRECTION ( 'NONE',  ( 0.6368676505102707219, 0.000000000000000000, 0.7709731485165535192 ) ) ;
#3552=ORIENTED_EDGE ( 'NONE', *, *, #9012, .F. ) ;
#3553=VERTEX_POINT ( 'NONE', #452 ) ;
#3554=CARTESIAN_POINT ( 'NONE',  ( -225.1241593668336236, -19.00000000000000000, 185.9653539489990521 ) ) ;
#3558=DIRECTION ( 'NONE',  ( 0.6368676505102709440, 0.000000000000000000, 0.7709731485165532971 ) ) ;
#3565=EDGE_LOOP ( 'NONE', ( #8340, #857, #6309, #886 ) ) ;
#3567=CARTESIAN_POINT ( 'NONE',  ( -185.9653539489998195, -19.00000000000000000, -225.1241593668329699 ) ) ;
#3570=DIRECTION ( 'NONE',  ( -0.000000000000000000, -1.000000000000000000, 0.000000000000000000 ) ) ;
#3575=CARTESIAN_POINT ( 'NONE',  ( 225.1241593668336236, -30.00000000000000000, -185.9653539489990521 ) ) ;
#3577=EDGE_CURVE ( 'NONE', #9318, #7702, #10974, .T. ) ;
#3581=AXIS2_PLACEMENT_3D ( 'NONE', #10022, #10280, #4951 ) ;
#3582=VECTOR ( 'NONE', #1272, 999.9999999999998863 ) ;
#3584=AXIS2_PLACEMENT_3D ( 'NONE', #12690, #11762, #3551 ) ;
#3594=AXIS2_PLACEMENT_3D ( 'NONE', #2099, #1107, #8381 ) ;
#3603=AXIS2_PLACEMENT_3D ( 'NONE', #7503, #11574, #6512 ) ;
#3604=DIRECTION ( 'NONE',  ( 0.6368676505102707219, 0.000000000000000000, 0.7709731485165535192 ) ) ;
#3605=PLANE ( 'NONE',  #2202 ) ;
#3616=DIRECTION ( 'NONE',  ( 0.7709731485165535192, -0.000000000000000000, -0.6368676505102707219 ) ) ;
#3617=ORIENTED_EDGE ( 'NONE', *, *, #5384, .F. ) ;
#3619=ORIENTED_EDGE ( 'NONE', *, *, #39, .F. ) ;
#3620=DIRECTION ( 'NONE',  ( -0.4503334343941556295, 0.7071067811865489050, -0.5451603414287969906 ) ) ;
#3631=ORIENTED_EDGE ( 'NONE', *, *, #5666, .F. ) ;
#3633=ORIENTED_EDGE ( 'NONE', *, *, #6003, .T. ) ;
#3635=LINE ( 'NONE', #7977, #11536 ) ;
#3639=AXIS2_PLACEMENT_3D ( 'NONE', #7110, #11375, #12303 ) ;
#3643=DIRECTION ( 'NONE',  ( -0.4503334343941556295, 0.7071067811865489050, -0.5451603414287969906 ) ) ;
#3644=CARTESIAN_POINT ( 'NONE',  ( 131.7449682071765835, -30.00000000000000000, -261.2053404739389180 ) ) ;
#3649=ORIENTED_EDGE ( 'NONE', *, *, #11496, .T. ) ;
#3651=DIRECTION ( 'NONE',  ( 0.000000000000000000, 1.000000000000000000, 0.000000000000000000 ) ) ;
#3652=DIRECTION ( 'NONE',  ( 0.6368676505102707219, 0.000000000000000000, 0.7709731485165536302 ) ) ;
#3656=DIRECTION ( 'NONE',  ( 0.6368676505102707219, 0.000000000000000000, 0.7709731485165535192 ) ) ;
#3668=ORIENTED_EDGE ( 'NONE', *, *, #11615, .T. ) ;
#3670=CARTESIAN_POINT ( 'NONE',  ( -159.9811538081799824, 20.00000000000000000, -193.6684549073582389 ) ) ;
#3671=CARTESIAN_POINT ( 'NONE',  ( 153.9282213272189495, -19.40000000000000213, 245.7765299597151341 ) ) ;
#3673=AXIS2_PLACEMENT_3D ( 'NONE', #12216, #4001, #9141 ) ;
#3678=DIRECTION ( 'NONE',  ( 0.4503334343941555740, 0.7071067811865490160, 0.5451603414287971017 ) ) ;
#3680=ORIENTED_EDGE ( 'NONE', *, *, #2691, .T. ) ;
#3682=CARTESIAN_POINT ( 'NONE',  ( -289.8128292627096130, -19.40000000000000213, 10.41748504886635907 ) ) ;
#3688=VERTEX_POINT ( 'NONE', #9038 ) ;
#3694=CARTESIAN_POINT ( 'NONE',  ( -171.9542656377731475, 0.000000000000000000, -208.1627500994694344 ) ) ;
#3698=AXIS2_PLACEMENT_3D ( 'NONE', #4332, #5338, #4395 ) ;
#3701=CARTESIAN_POINT ( 'NONE',  ( 0.000000000000000000, 0.000000000000000000, 0.000000000000000000 ) ) ;
#3703=ORIENTED_EDGE ( 'NONE', *, *, #6003, .F. ) ;
#3704=ADVANCED_FACE ( 'NONE', ( #1300 ), #3515, .T. ) ;
#3705=DIRECTION ( 'NONE',  ( -0.000000000000000000, -1.000000000000000000, 0.000000000000000000 ) ) ;
#3709=CARTESIAN_POINT ( 'NONE',  ( -189.4681260268063170, -19.00000000000000000, -229.3645116836740385 ) ) ;
#3715=ORIENTED_EDGE ( 'NONE', *, *, #5156, .F. ) ;
#3720=ORIENTED_EDGE ( 'NONE', *, *, #10099, .F. ) ;
#3726=CIRCLE ( 'NONE', #3505, 305.0000000000000000 ) ;
#3748=EDGE_CURVE ( 'NONE', #5508, #8628, #4227, .T. ) ;
#3750=ORIENTED_EDGE ( 'NONE', *, *, #11172, .F. ) ;
#3755=DIRECTION ( 'NONE',  ( 0.6368676505102700558, 0.000000000000000000, 0.7709731485165541853 ) ) ;
#3759=EDGE_LOOP ( 'NONE', ( #4111, #11282 ) ) ;
#3760=DIRECTION ( 'NONE',  ( -0.000000000000000000, -1.000000000000000000, 0.000000000000000000 ) ) ;
#3763=ORIENTED_EDGE ( 'NONE', *, *, #11496, .F. ) ;
#3779=ORIENTED_EDGE ( 'NONE', *, *, #8425, .T. ) ;
#3784=CARTESIAN_POINT ( 'NONE',  ( -290.6841825403030839, -19.00000000000000000, -27.68945685411394919 ) ) ;
#3786=EDGE_CURVE ( 'NONE', #9988, #8945, #8433, .T. ) ;
#3787=FACE_OUTER_BOUND ( 'NONE', #5863, .T. ) ;
#3788=CARTESIAN_POINT ( 'NONE',  ( 149.7885815989021694, -18.00000000000000000, 240.7652044943575333 ) ) ;
#3790=CIRCLE ( 'NONE', #1888, 251.8333333333299606 ) ;
#3791=CARTESIAN_POINT ( 'NONE',  ( 165.3358371128620377, -2.772967769358684720, 200.1506762031205255 ) ) ;
#3792=AXIS2_PLACEMENT_3D ( 'NONE', #752, #4802, #11071 ) ;
#3793=EDGE_CURVE ( 'NONE', #6648, #2275, #5221, .T. ) ;
#3809=DIRECTION ( 'NONE',  ( -0.000000000000000000, -1.000000000000000000, 0.000000000000000000 ) ) ;
#3814=ORIENTED_EDGE ( 'NONE', *, *, #12845, .T. ) ;
#3817=EDGE_LOOP ( 'NONE', ( #5317, #11371 ) ) ;
#3823=EDGE_CURVE ( 'NONE', #8455, #10237, #8242, .T. ) ;
#3828=ORIENTED_EDGE ( 'NONE', *, *, #9998, .F. ) ;
#3829=CARTESIAN_POINT ( 'NONE',  ( -159.3442861576697283, -29.00000000000000000, -192.8974817588416499 ) ) ;
#3830=ORIENTED_EDGE ( 'NONE', *, *, #12015, .T. ) ;
#3832=ORIENTED_EDGE ( 'NONE', *, *, #6725, .T. ) ;
#3836=CARTESIAN_POINT ( 'NONE',  ( -293.0608542803120145, -30.00000000000000000, 6.485521991431936861 ) ) ;
#3845=CARTESIAN_POINT ( 'NONE',  ( -159.6627199829248696, -25.00000000000000000, -193.2829683330999728 ) ) ;
#3846=EDGE_LOOP ( 'NONE', ( #6564, #7607, #10496, #11228 ) ) ;
#3853=CARTESIAN_POINT ( 'NONE',  ( -289.8128292627096130, -28.60000000000000142, 10.41748504886635907 ) ) ;
#3860=LINE ( 'NONE', #6007, #3496 ) ;
#3862=EDGE_CURVE ( 'NONE', #11555, #2690, #7053, .T. ) ;
#3866=EDGE_LOOP ( 'NONE', ( #8483, #5014, #9616, #3680 ) ) ;
#3867=ORIENTED_EDGE ( 'NONE', *, *, #9567, .T. ) ;
#3868=CIRCLE ( 'NONE', #7283, 5.500000000000007994 ) ;
#3869=DIRECTION ( 'NONE',  ( 0.6368676505102707219, 0.000000000000000000, 0.7709731485165535192 ) ) ;
#3871=EDGE_CURVE ( 'NONE', #2079, #11697, #10545, .T. ) ;
#3872=CIRCLE ( 'NONE', #5579, 250.1999999999999602 ) ;
#3874=LINE ( 'NONE', #2865, #711 ) ;
#3883=ORIENTED_EDGE ( 'NONE', *, *, #1321, .F. ) ;
#3893=( NAMED_UNIT ( * ) PLANE_ANGLE_UNIT ( ) SI_UNIT ( $, .RADIAN. ) );
#3897=AXIS2_PLACEMENT_3D ( 'NONE', #3554, #5368, #7627 ) ;
#3900=AXIS2_PLACEMENT_3D ( 'NONE', #5360, #9430, #2483 ) ;
#3912=EDGE_LOOP ( 'NONE', ( #9683, #971, #10820, #232 ) ) ;
#3918=ORIENTED_EDGE ( 'NONE', *, *, #10806, .F. ) ;
#3926=CONICAL_SURFACE ( 'NONE', #9669, 6.500000000000000888, 0.7853981633974617127 ) ;
#3932=ORIENTED_EDGE ( 'NONE', *, *, #11867, .F. ) ;
#3933=VERTEX_POINT ( 'NONE', #4610 ) ;
#3935=CARTESIAN_POINT ( 'NONE',  ( -185.9653539489998195, -29.00000000000000000, -225.1241593668329699 ) ) ;
#3940=EDGE_CURVE ( 'NONE', #9649, #169, #9615, .T. ) ;
#3944=TOROIDAL_SURFACE ( 'NONE', #1610, 261.5294117647060261, 2.000000000000000000 ) ;
#3953=DIRECTION ( 'NONE',  ( 0.4503334343941595153, -0.7071067811865431318, 0.5451603414288016536 ) ) ;
#3955=CARTESIAN_POINT ( 'NONE',  ( -159.3442861576697283, 19.00000000000000000, -192.8974817588417352 ) ) ;
#3960=ORIENTED_EDGE ( 'NONE', *, *, #2991, .T. ) ;
#3962=DIRECTION ( 'NONE',  ( -0.6368676505102696117, 0.000000000000000000, -0.7709731485165545184 ) ) ;
#3966=DIRECTION ( 'NONE',  ( -0.000000000000000000, -1.000000000000000000, 0.000000000000000000 ) ) ;
#3967=DIRECTION ( 'NONE',  ( 0.4503334343941555740, 0.7071067811865490160, 0.5451603414287971017 ) ) ;
#3975=VERTEX_POINT ( 'NONE', #1495 ) ;
#3976=DIRECTION ( 'NONE',  ( -0.000000000000000000, -1.000000000000000000, 0.000000000000000000 ) ) ;
#3981=DIRECTION ( 'NONE',  ( -0.000000000000000000, -1.000000000000000000, 0.000000000000000000 ) ) ;
#3985=EDGE_CURVE ( 'NONE', #11069, #169, #12737, .T. ) ;
#3987=ADVANCED_FACE ( 'NONE', ( #11701 ), #10613, .F. ) ;
#3994=ORIENTED_EDGE ( 'NONE', *, *, #12176, .F. ) ;
#3995=DIRECTION ( 'NONE',  ( 0.4503334343941626794, -0.7071067811865380248, 0.5451603414288055394 ) ) ;
#3999=CARTESIAN_POINT ( 'NONE',  ( -181.8257142206830679, -30.00000000000000000, -220.1128339014753692 ) ) ;
#4001=DIRECTION ( 'NONE',  ( -0.000000000000000000, -1.000000000000000000, 0.000000000000000000 ) ) ;
#4006=DIRECTION ( 'NONE',  ( -0.6368676505102708330, 0.000000000000000000, -0.7709731485165536302 ) ) ;
#4008=ORIENTED_EDGE ( 'NONE', *, *, #12259, .F. ) ;
#4010=ORIENTED_EDGE ( 'NONE', *, *, #6649, .F. ) ;
#4011=EDGE_CURVE ( 'NONE', #11136, #8469, #4483, .T. ) ;
#4012=CIRCLE ( 'NONE', #9989, 5.500000000000007994 ) ;
#4015=DIRECTION ( 'NONE',  ( -0.000000000000000000, -1.000000000000000000, 0.000000000000000000 ) ) ;
#4017=VECTOR ( 'NONE', #4212, 1000.000000000000000 ) ;
#4018=DIRECTION ( 'NONE',  ( 0.6368676505102716101, 0.000000000000000000, 0.7709731485165527420 ) ) ;
#4019=AXIS2_PLACEMENT_3D ( 'NONE', #12858, #3651, #11859 ) ;
#4024=AXIS2_PLACEMENT_3D ( 'NONE', #9043, #3159, #7244 ) ;
#4026=FACE_OUTER_BOUND ( 'NONE', #6436, .T. ) ;
#4032=CIRCLE ( 'NONE', #5315, 6.500000000000005329 ) ;
#4033=DIRECTION ( 'NONE',  ( 0.6368676505102707219, 0.000000000000000000, 0.7709731485165535192 ) ) ;
#4038=EDGE_CURVE ( 'NONE', #1970, #4613, #12536, .T. ) ;
#4039=CARTESIAN_POINT ( 'NONE',  ( 294.1869546181097235, -19.00000000000000000, 31.92980917095290749 ) ) ;
#4062=VERTEX_POINT ( 'NONE', #8567 ) ;
#4064=EDGE_CURVE ( 'NONE', #2618, #4412, #10402, .T. ) ;
#4068=DIRECTION ( 'NONE',  ( 0.7709731485165535192, 0.000000000000000000, -0.6368676505102707219 ) ) ;
#4071=DIRECTION ( 'NONE',  ( -0.000000000000000000, -1.000000000000000000, 0.000000000000000000 ) ) ;
#4077=VERTEX_POINT ( 'NONE', #6567 ) ;
#4081=ADVANCED_FACE ( 'NONE', ( #2426 ), #12956, .F. ) ;
#4083=EDGE_CURVE ( 'NONE', #9366, #327, #6701, .T. ) ;
#4084=FACE_OUTER_BOUND ( 'NONE', #11700, .T. ) ;
#4086=CIRCLE ( 'NONE', #8774, 6.500000000000005329 ) ;
#4089=AXIS2_PLACEMENT_3D ( 'NONE', #3100, #7176, #6317 ) ;
#4091=ADVANCED_FACE ( 'NONE', ( #1561 ), #565, .F. ) ;
#4096=DIRECTION ( 'NONE',  ( 0.6368676505102707219, 0.000000000000000000, 0.7709731485165536302 ) ) ;
#4098=CIRCLE ( 'NONE', #6020, 259.6078431372549744 ) ;
#4099=CIRCLE ( 'NONE', #7094, 5.500000000000015099 ) ;
#4106=DIRECTION ( 'NONE',  ( 0.6368676505102698338, 0.000000000000000000, 0.7709731485165542964 ) ) ;
#4107=EDGE_CURVE ( 'NONE', #3688, #9318, #1680, .T. ) ;
#4111=ORIENTED_EDGE ( 'NONE', *, *, #11687, .F. ) ;
#4117=CARTESIAN_POINT ( 'NONE',  ( 160.6180214586902366, -11.79660968244695951, 194.4394280558747994 ) ) ;
#4122=FACE_OUTER_BOUND ( 'NONE', #3489, .T. ) ;
#4126=CARTESIAN_POINT ( 'NONE',  ( 24.18668477630848557, -30.00000000000000000, -294.9245348571437262 ) ) ;
#4135=FACE_OUTER_BOUND ( 'NONE', #12691, .T. ) ;
#4140=CARTESIAN_POINT ( 'NONE',  ( 161.8917567597108018, -22.00000000000000000, 195.9813743529078920 ) ) ;
#4144=ORIENTED_EDGE ( 'NONE', *, *, #12991, .F. ) ;
#4145=CARTESIAN_POINT ( 'NONE',  ( -0.000000000000000000, -11.79660968244695951, 0.000000000000000000 ) ) ;
#4150=CYLINDRICAL_SURFACE ( 'NONE', #12112, 5.500000000000015099 ) ;
#4151=DIRECTION ( 'NONE',  ( -0.7709731485165536302, 0.000000000000000000, 0.6368676505102706109 ) ) ;
#4158=ADVANCED_FACE ( 'NONE', ( #6895 ), #8884, .F. ) ;
#4160=ORIENTED_EDGE ( 'NONE', *, *, #4320, .F. ) ;
#4161=DIRECTION ( 'NONE',  ( -0.000000000000000000, -1.000000000000000000, 0.000000000000000000 ) ) ;
#4162=ORIENTED_EDGE ( 'NONE', *, *, #8682, .T. ) ;
#4164=ORIENTED_EDGE ( 'NONE', *, *, #39, .T. ) ;
#4175=ORIENTED_EDGE ( 'NONE', *, *, #12991, .T. ) ;
#4176=ORIENTED_EDGE ( 'NONE', *, *, #5583, .T. ) ;
#4180=VERTEX_POINT ( 'NONE', #764 ) ;
#4192=DIRECTION ( 'NONE',  ( -0.000000000000000000, -1.000000000000000000, 0.000000000000000000 ) ) ;
#4194=ORIENTED_EDGE ( 'NONE', *, *, #1434, .T. ) ;
#4201=ADVANCED_FACE ( 'NONE', ( #3136 ), #4642, .F. ) ;
#4212=DIRECTION ( 'NONE',  ( -0.4503334343941575724, 0.7071067811865460184, -0.5451603414287993221 ) ) ;
#4216=DIRECTION ( 'NONE',  ( -0.000000000000000000, -1.000000000000000000, 0.000000000000000000 ) ) ;
#4219=ORIENTED_EDGE ( 'NONE', *, *, #3940, .F. ) ;
#4224=AXIS2_PLACEMENT_3D ( 'NONE', #10925, #7997, #12057 ) ;
#4227=LINE ( 'NONE', #5364, #7567 ) ;
#4228=ORIENTED_EDGE ( 'NONE', *, *, #9934, .F. ) ;
#4230=CIRCLE ( 'NONE', #4019, 250.1999999999999602 ) ;
#4231=EDGE_CURVE ( 'NONE', #10245, #10624, #9131, .T. ) ;
#4234=CARTESIAN_POINT ( 'NONE',  ( -0.000000000000000000, -30.00000000000000000, 0.000000000000000000 ) ) ;
#4243=ORIENTED_EDGE ( 'NONE', *, *, #10480, .T. ) ;
#4252=CARTESIAN_POINT ( 'NONE',  ( 159.3442861576696714, -11.79660968244695951, 192.8974817588417068 ) ) ;
#4258=CARTESIAN_POINT ( 'NONE',  ( 160.3845033201290846, -9.830508068730530624, 194.1567379013694392 ) ) ;
#4264=CARTESIAN_POINT ( 'NONE',  ( 23.54981712579821362, -30.00000000000000000, -295.6955080056602583 ) ) ;
#4274=VERTEX_POINT ( 'NONE', #4343 ) ;
#4276=DIRECTION ( 'NONE',  ( -0.000000000000000000, -1.000000000000000000, 0.000000000000000000 ) ) ;
#4277=DIRECTION ( 'NONE',  ( 0.6368676505102716101, 0.000000000000000000, 0.7709731485165527420 ) ) ;
#4278=EDGE_LOOP ( 'NONE', ( #6101, #8536 ) ) ;
#4282=DIRECTION ( 'NONE',  ( -0.000000000000000000, -1.000000000000000000, 0.000000000000000000 ) ) ;
#4289=ORIENTED_EDGE ( 'NONE', *, *, #10186, .F. ) ;
#4292=DIRECTION ( 'NONE',  ( -0.000000000000000000, -1.000000000000000000, 0.000000000000000000 ) ) ;
#4294=ORIENTED_EDGE ( 'NONE', *, *, #4821, .T. ) ;
#4295=DIRECTION ( 'NONE',  ( -0.000000000000000000, -1.000000000000000000, 0.000000000000000000 ) ) ;
#4297=DIRECTION ( 'NONE',  ( 0.6368676505102716101, 0.000000000000000000, 0.7709731485165527420 ) ) ;
#4299=LINE ( 'NONE', #6904, #945 ) ;
#4305=CARTESIAN_POINT ( 'NONE',  ( -194.2446334056326123, -19.00000000000000000, -235.1468102975487682 ) ) ;
#4306=AXIS2_PLACEMENT_3D ( 'NONE', #757, #685, #619 ) ;
#4309=FACE_OUTER_BOUND ( 'NONE', #3537, .T. ) ;
#4310=CARTESIAN_POINT ( 'NONE',  ( -160.3845033201972115, 9.830508068689120194, -194.1567379014518906 ) ) ;
#4320=EDGE_CURVE ( 'NONE', #2539, #11730, #3872, .T. ) ;
#4332=CARTESIAN_POINT ( 'NONE',  ( -0.000000000000000000, -2.772967769358684720, 0.000000000000000000 ) ) ;
#4337=CIRCLE ( 'NONE', #9459, 10.00000000000000178 ) ;
#4343=CARTESIAN_POINT ( 'NONE',  ( 189.4681260268079086, -19.00000000000000000, 229.3645116836727311 ) ) ;
#4345=ORIENTED_EDGE ( 'NONE', *, *, #6118, .T. ) ;
#4346=CONICAL_SURFACE ( 'NONE', #8822, 6.500000000000005329, 0.7853981633974547183 ) ;
#4348=DIRECTION ( 'NONE',  ( 0.000000000000000000, 1.000000000000000000, 0.000000000000000000 ) ) ;
#4351=EDGE_CURVE ( 'NONE', #9382, #4180, #11332, .T. ) ;
#4357=AXIS2_PLACEMENT_3D ( 'NONE', #9929, #8003, #13000 ) ;
#4360=ORIENTED_EDGE ( 'NONE', *, *, #11711, .T. ) ;
#4362=ORIENTED_EDGE ( 'NONE', *, *, #6458, .F. ) ;
#4372=ORIENTED_EDGE ( 'NONE', *, *, #3287, .T. ) ;
#4375=ORIENTED_EDGE ( 'NONE', *, *, #4966, .T. ) ;
#4387=DIRECTION ( 'NONE',  ( 0.000000000000000000, 1.000000000000000000, 0.000000000000000000 ) ) ;
#4388=ORIENTED_EDGE ( 'NONE', *, *, #8609, .F. ) ;
#4391=DIRECTION ( 'NONE',  ( 0.6368676505102707219, 0.000000000000000000, 0.7709731485165535192 ) ) ;
#4395=DIRECTION ( 'NONE',  ( -0.6368676505102708330, 0.000000000000000000, -0.7709731485165536302 ) ) ;
#4399=CARTESIAN_POINT ( 'NONE',  ( -0.000000000000000000, -25.00000000000000000, 0.000000000000000000 ) ) ;
#4401=ORIENTED_EDGE ( 'NONE', *, *, #12873, .T. ) ;
#4402=EDGE_LOOP ( 'NONE', ( #12692, #631, #41, #11347 ) ) ;
#4404=CARTESIAN_POINT ( 'NONE',  ( -159.6627199829249264, -22.00000000000000000, -193.2829683330999728 ) ) ;
#4412=VERTEX_POINT ( 'NONE', #2408 ) ;
#4416=EDGE_CURVE ( 'NONE', #9350, #12436, #6447, .T. ) ;
#4418=ORIENTED_EDGE ( 'NONE', *, *, #5760, .T. ) ;
#4419=VERTEX_POINT ( 'NONE', #352 ) ;
#4422=DIRECTION ( 'NONE',  ( -0.6368676505102706109, 0.000000000000000000, -0.7709731485165535192 ) ) ;
#4425=DIRECTION ( 'NONE',  ( -0.000000000000000000, -1.000000000000000000, 0.000000000000000000 ) ) ;
#4427=AXIS2_PLACEMENT_3D ( 'NONE', #8487, #9483, #7674 ) ;
#4430=ORIENTED_EDGE ( 'NONE', *, *, #11828, .T. ) ;
#4431=CARTESIAN_POINT ( 'NONE',  ( 225.1241593668336236, -19.00000000000000000, -185.9653539489990521 ) ) ;
#4432=ORIENTED_EDGE ( 'NONE', *, *, #6458, .T. ) ;
#4435=CARTESIAN_POINT ( 'NONE',  ( -0.000000000000000000, -3.327561323230905366, 0.000000000000000000 ) ) ;
#4438=CIRCLE ( 'NONE', #3161, 305.0000000000000000 ) ;
#4441=LINE ( 'NONE', #8525, #3173 ) ;
#4442=CARTESIAN_POINT ( 'NONE',  ( 0.000000000000000000, 20.00000000000000000, 0.000000000000000000 ) ) ;
#4444=CIRCLE ( 'NONE', #9555, 6.500000000000000888 ) ;
#4445=DIRECTION ( 'NONE',  ( 0.6368676505102716101, 0.000000000000000000, 0.7709731485165527420 ) ) ;
#4449=AXIS2_PLACEMENT_3D ( 'NONE', #9971, #9838, #6657 ) ;
#4453=DIRECTION ( 'NONE',  ( -0.6368676505102698338, 0.000000000000000000, -0.7709731485165542964 ) ) ;
#4456=VECTOR ( 'NONE', #8316, 1000.000000000000114 ) ;
#4458=VECTOR ( 'NONE', #7518, 999.9999999999998863 ) ;
#4462=CARTESIAN_POINT ( 'NONE',  ( 193.6077657551222444, -30.00000000000000000, 234.3758371490322929 ) ) ;
#4463=EDGE_CURVE ( 'NONE', #2690, #11555, #10486, .T. ) ;
#4464=PRODUCT ( 'External Heavy Duty Rotating Flange Ring', 'External Heavy Duty Rotating Flange Ring', '', ( #4511 ) ) ;
#4465=DIRECTION ( 'NONE',  ( -0.000000000000000000, -1.000000000000000000, 0.000000000000000000 ) ) ;
#4466=VERTEX_POINT ( 'NONE', #8943 ) ;
#4469=LINE ( 'NONE', #11622, #2519 ) ;
#4470=FACE_BOUND ( 'NONE', #4278, .T. ) ;
#4471=CONICAL_SURFACE ( 'NONE', #8961, 6.500000000000005329, 0.7853981633974476129 ) ;
#4482=ORIENTED_EDGE ( 'NONE', *, *, #3491, .T. ) ;
#4483=LINE ( 'NONE', #10623, #6371 ) ;
#4484=ORIENTED_EDGE ( 'NONE', *, *, #4463, .F. ) ;
#4486=LINE ( 'NONE', #11573, #2615 ) ;
#4489=ADVANCED_FACE ( 'NONE', ( #12009 ), #10054, .T. ) ;
#4493=AXIS2_PLACEMENT_3D ( 'NONE', #1105, #1939, #4033 ) ;
#4497=CARTESIAN_POINT ( 'NONE',  ( -286.5445428119863323, -30.00000000000000000, -22.67813138875635204 ) ) ;
#4498=VERTEX_POINT ( 'NONE', #1871 ) ;
#4500=CARTESIAN_POINT ( 'NONE',  ( -0.000000000000000000, -1.848645179577135034, 0.000000000000000000 ) ) ;
#4501=CARTESIAN_POINT ( 'NONE',  ( 132.6365829178909621, -30.00000000000000000, -260.1259780660157048 ) ) ;
#4503=CARTESIAN_POINT ( 'NONE',  ( 195.9813743529078920, -25.00000000000000000, -161.8917567597108018 ) ) ;
#4509=AXIS2_PLACEMENT_3D ( 'NONE', #4540, #5681, #1751 ) ;
#4511=PRODUCT_CONTEXT ( 'NONE', #914, 'mechanical' ) ;
#4513=CARTESIAN_POINT ( 'NONE',  ( -189.4681260268063170, -19.00000000000000000, -229.3645116836740385 ) ) ;
#4518=CARTESIAN_POINT ( 'NONE',  ( 159.6627199829248980, -22.00000000000000000, 193.2829683331000012 ) ) ;
#4529=CIRCLE ( 'NONE', #4963, 2.500000000000025313 ) ;
#4530=CLOSED_SHELL ( 'NONE', ( #8249, #8248, #7368, #5086, #3507, #10945, #4936, #4081, #6467, #5477, #10240, #2123, #6318, #7662, #6147, #6484, #4201, #10961, #8527, #5620, #5327, #8026, #1086, #6365, #10127, #3410, #5540, #8719, #7463, #11753, #8484, #11030, #7267, #9861, #276, #6771, #1255, #7630, #11613, #11130, #10515, #8032, #3704, #11494, #7218, #2294, #9504, #3987, #8909, #7934, #445, #702, #1494, #6296, #10387, #1398, #7621, #4158, #4688, #9550, #2708, #4813, #4489, #11973, #1154, #8883, #11278, #8348, #6163, #385, #2671, #4835, #9778, #11379, #11527, #11258, #9078, #7528, #12163, #11541, #1803, #8836, #5406, #8856, #10773, #9053, #10862, #1199, #9174, #11049, #1963, #11003, #3359, #1109, #1137, #1748, #6621, #12349, #7144, #1346, #2837, #7214, #66, #1652, #4091, #1228, #11797, #2973, #177, #11785, #418 ) ) ;
#4531=CARTESIAN_POINT ( 'NONE',  ( 171.9542656377731191, 0.000000000000000000, 208.1627500994694628 ) ) ;
#4533=DIRECTION ( 'NONE',  ( -0.000000000000000000, -1.000000000000000000, 0.000000000000000000 ) ) ;
#4534=ORIENTED_EDGE ( 'NONE', *, *, #1723, .T. ) ;
#4540=CARTESIAN_POINT ( 'NONE',  ( -290.6841825403030839, -30.00000000000000000, -27.68945685411394919 ) ) ;
#4548=ORIENTED_EDGE ( 'NONE', *, *, #5095, .F. ) ;
#4550=ORIENTED_EDGE ( 'NONE', *, *, #6226, .F. ) ;
#4554=EDGE_CURVE ( 'NONE', #11136, #5893, #12818, .T. ) ;
#4558=AXIS2_PLACEMENT_3D ( 'NONE', #12347, #7404, #11477 ) ;
#4559=DIRECTION ( 'NONE',  ( 0.6368676505102716101, 0.000000000000000000, 0.7709731485165527420 ) ) ;
#4564=DIRECTION ( 'NONE',  ( -0.6368676505102696117, 0.000000000000000000, -0.7709731485165545184 ) ) ;
#4572=CIRCLE ( 'NONE', #6088, 259.6078431372534396 ) ;
#4581=DIRECTION ( 'NONE',  ( 0.6368676505102709440, 0.000000000000000000, 0.7709731485165532971 ) ) ;
#4583=CIRCLE ( 'NONE', #12047, 5.100000000000003197 ) ;
#4585=DIRECTION ( 'NONE',  ( 0.000000000000000000, 1.000000000000000000, 0.000000000000000000 ) ) ;
#4586=DIRECTION ( 'NONE',  ( 0.000000000000000000, 1.000000000000000000, 0.000000000000000000 ) ) ;
#4596=ORIENTED_EDGE ( 'NONE', *, *, #4083, .F. ) ;
#4599=DIRECTION ( 'NONE',  ( 0.6368676505102707219, 0.000000000000000000, 0.7709731485165535192 ) ) ;
#4602=CARTESIAN_POINT ( 'NONE',  ( -161.8917567597108587, -22.00000000000000000, -195.9813743529078636 ) ) ;
#4607=ORIENTED_EDGE ( 'NONE', *, *, #11867, .T. ) ;
#4610=CARTESIAN_POINT ( 'NONE',  ( -171.9542656377731475, 19.00000000000000000, -208.1627500994694344 ) ) ;
#4613=VERTEX_POINT ( 'NONE', #5121 ) ;
#4615=DIRECTION ( 'NONE',  ( -0.000000000000000000, -1.000000000000000000, 0.000000000000000000 ) ) ;
#4618=CARTESIAN_POINT ( 'NONE',  ( -290.6841825403030839, -29.00000000000000000, -27.68945685411394919 ) ) ;
#4622=CYLINDRICAL_SURFACE ( 'NONE', #1785, 250.1999999999999602 ) ;
#4623=ORIENTED_EDGE ( 'NONE', *, *, #3273, .T. ) ;
#4631=CARTESIAN_POINT ( 'NONE',  ( 294.8238222686199492, -18.00000000000000000, 32.70078231946946090 ) ) ;
#4634=DIRECTION ( 'NONE',  ( -0.000000000000000000, -1.000000000000000000, 0.000000000000000000 ) ) ;
#4636=CARTESIAN_POINT ( 'NONE',  ( 27.68945685411497593, -30.00000000000000000, -290.6841825403026291 ) ) ;
#4637=EDGE_LOOP ( 'NONE', ( #12884, #3187, #3867, #9831 ) ) ;
#4640=ORIENTED_EDGE ( 'NONE', *, *, #8577, .T. ) ;
#4642=CONICAL_SURFACE ( 'NONE', #9757, 5.500000000000007994, 0.7853981633974461696 ) ;
#4648=CIRCLE ( 'NONE', #8071, 6.500000000000005329 ) ;
#4651=DIRECTION ( 'NONE',  ( 0.7709731485165535192, 0.000000000000000000, -0.6368676505102707219 ) ) ;
#4654=LINE ( 'NONE', #8734, #7501 ) ;
#4659=DIRECTION ( 'NONE',  ( 0.6368676505102716101, 0.000000000000000000, 0.7709731485165527420 ) ) ;
#4661=VERTEX_POINT ( 'NONE', #3119 ) ;
#4662=EDGE_LOOP ( 'NONE', ( #10223, #3763, #6778, #5461 ) ) ;
#4663=CIRCLE ( 'NONE', #3603, 6.500000000000005329 ) ;
#4664=DIRECTION ( 'NONE',  ( -0.000000000000000000, -1.000000000000000000, 0.000000000000000000 ) ) ;
#4667=EDGE_CURVE ( 'NONE', #3975, #900, #1967, .T. ) ;
#4672=LINE ( 'NONE', #7808, #1777 ) ;
#4673=AXIS2_PLACEMENT_3D ( 'NONE', #8606, #10660, #1534 ) ;
#4674=EDGE_LOOP ( 'NONE', ( #10313, #5793 ) ) ;
#4678=ORIENTED_EDGE ( 'NONE', *, *, #6647, .F. ) ;
#4679=EDGE_LOOP ( 'NONE', ( #9829, #8393, #8109, #1563 ) ) ;
#4687=LINE ( 'NONE', #10069, #2449 ) ;
#4688=ADVANCED_FACE ( 'NONE', ( #9332 ), #2108, .F. ) ;
#4689=CARTESIAN_POINT ( 'NONE',  ( 150.6801963096165764, -28.60000000000000142, 241.8445669022807181 ) ) ;
#4690=DIRECTION ( 'NONE',  ( 0.000000000000000000, 1.000000000000000000, 0.000000000000000000 ) ) ;
#4692=ORIENTED_EDGE ( 'NONE', *, *, #5816, .T. ) ;
#4702=AXIS2_PLACEMENT_3D ( 'NONE', #1236, #1433, #3350 ) ;
#4704=ORIENTED_EDGE ( 'NONE', *, *, #9961, .F. ) ;
#4705=CYLINDRICAL_SURFACE ( 'NONE', #5650, 5.500000000000015099 ) ;
#4707=EDGE_LOOP ( 'NONE', ( #1415, #4010, #3087, #676 ) ) ;
#4714=CARTESIAN_POINT ( 'NONE',  ( -228.6269314446401211, -30.00000000000000000, 181.7250016321579835 ) ) ;
#4721=FACE_OUTER_BOUND ( 'NONE', #2554, .T. ) ;
#4735=AXIS2_PLACEMENT_3D ( 'NONE', #3198, #6346, #5271 ) ;
#4739=FACE_OUTER_BOUND ( 'NONE', #8566, .T. ) ;
#4743=ORIENTED_EDGE ( 'NONE', *, *, #7766, .T. ) ;
#4747=CONICAL_SURFACE ( 'NONE', #10922, 5.500000000000007994, 0.7853981633974461696 ) ;
#4755=DIRECTION ( 'NONE',  ( -0.000000000000000000, -1.000000000000000000, 0.000000000000000000 ) ) ;
#4756=CARTESIAN_POINT ( 'NONE',  ( -220.9845196385168435, -30.00000000000000000, 190.9766794143566528 ) ) ;
#4760=AXIS2_PLACEMENT_3D ( 'NONE', #12597, #7533, #11926 ) ;
#4761=FACE_OUTER_BOUND ( 'NONE', #5926, .T. ) ;
#4766=CIRCLE ( 'NONE', #7331, 6.500000000000005329 ) ;
#4768=CARTESIAN_POINT ( 'NONE',  ( 153.9282213272189495, -19.40000000000000213, 245.7765299597151341 ) ) ;
#4769=DIRECTION ( 'NONE',  ( -0.6368676505102707219, 0.000000000000000000, -0.7709731485165535192 ) ) ;
#4770=CIRCLE ( 'NONE', #11161, 6.500000000000026645 ) ;
#4772=EDGE_CURVE ( 'NONE', #2640, #10885, #4444, .T. ) ;
#4783=ORIENTED_EDGE ( 'NONE', *, *, #12471, .T. ) ;
#4787=LINE ( 'NONE', #667, #9724 ) ;
#4788=CIRCLE ( 'NONE', #12252, 2.000000000000000444 ) ;
#4802=DIRECTION ( 'NONE',  ( -0.000000000000000000, -1.000000000000000000, 0.000000000000000000 ) ) ;
#4807=CARTESIAN_POINT ( 'NONE',  ( -185.9653539489998195, -19.00000000000000000, -225.1241593668329699 ) ) ;
#4812=ORIENTED_EDGE ( 'NONE', *, *, #9998, .T. ) ;
#4813=ADVANCED_FACE ( 'NONE', ( #10529 ), #10193, .F. ) ;
#4814=DIRECTION ( 'NONE',  ( 0.4503334343941555740, 0.7071067811865490160, 0.5451603414287971017 ) ) ;
#4821=EDGE_CURVE ( 'NONE', #7406, #11365, #1047, .T. ) ;
#4822=ORIENTED_EDGE ( 'NONE', *, *, #8129, .T. ) ;
#4824=ORIENTED_EDGE ( 'NONE', *, *, #8325, .F. ) ;
#4835=ADVANCED_FACE ( 'NONE', ( #266 ), #9764, .F. ) ;
#4843=EDGE_LOOP ( 'NONE', ( #1526, #562, #4812, #4822 ) ) ;
#4846=ORIENTED_EDGE ( 'NONE', *, *, #10380, .F. ) ;
#4851=DIRECTION ( 'NONE',  ( 0.000000000000000000, 1.000000000000000000, 0.000000000000000000 ) ) ;
#4856=CARTESIAN_POINT ( 'NONE',  ( 157.1762463448213225, -28.60000000000000142, 249.7084930171495785 ) ) ;
#4858=VECTOR ( 'NONE', #5965, 1000.000000000000000 ) ;
#4860=CARTESIAN_POINT ( 'NONE',  ( -0.000000000000000000, -30.00000000000000000, 0.000000000000000000 ) ) ;
#4861=CIRCLE ( 'NONE', #3792, 250.1999999999999602 ) ;
#4862=AXIS2_PLACEMENT_3D ( 'NONE', #6948, #5402, #12529 ) ;
#4865=AXIS2_PLACEMENT_3D ( 'NONE', #3682, #2552, #500 ) ;
#4868=EDGE_LOOP ( 'NONE', ( #1231, #12804, #12420, #1672 ) ) ;
#4871=FACE_BOUND ( 'NONE', #3759, .T. ) ;
#4874=FACE_OUTER_BOUND ( 'NONE', #11957, .T. ) ;
#4877=DIRECTION ( 'NONE',  ( 0.6368676505102707219, 0.000000000000000000, 0.7709731485165536302 ) ) ;
#4878=CIRCLE ( 'NONE', #10629, 254.1999999999999886 ) ;
#4888=FACE_OUTER_BOUND ( 'NONE', #2410, .T. ) ;
#4893=CARTESIAN_POINT ( 'NONE',  ( 287.1814104624967854, -19.00000000000000000, 23.44910453727081290 ) ) ;
#4894=EDGE_CURVE ( 'NONE', #8752, #9436, #12593, .T. ) ;
#4896=EDGE_LOOP ( 'NONE', ( #2050, #9520, #7869, #5491 ) ) ;
#4898=ORIENTED_EDGE ( 'NONE', *, *, #7024, .F. ) ;
#4900=ORIENTED_EDGE ( 'NONE', *, *, #12793, .F. ) ;
#4904=FACE_OUTER_BOUND ( 'NONE', #10983, .T. ) ;
#4911=ORIENTED_EDGE ( 'NONE', *, *, #3985, .T. ) ;
#4914=ORIENTED_EDGE ( 'NONE', *, *, #10186, .T. ) ;
#4915=ORIENTED_EDGE ( 'NONE', *, *, #12321, .T. ) ;
#4917=ORIENTED_EDGE ( 'NONE', *, *, #1252, .F. ) ;
#4924=AXIS2_PLACEMENT_3D ( 'NONE', #10976, #6845, #2038 ) ;
#4936=ADVANCED_FACE ( 'NONE', ( #5862 ), #8932, .F. ) ;
#4950=LINE ( 'NONE', #9028, #7003 ) ;
#4951=DIRECTION ( 'NONE',  ( 0.6368676505102700558, 0.000000000000000000, 0.7709731485165541853 ) ) ;
#4954=AXIS2_PLACEMENT_3D ( 'NONE', #5374, #11578, #2299 ) ;
#4956=DIRECTION ( 'NONE',  ( -0.000000000000000000, -1.000000000000000000, 0.000000000000000000 ) ) ;
#4963=AXIS2_PLACEMENT_3D ( 'NONE', #3387, #8473, #9524 ) ;
#4966=EDGE_CURVE ( 'NONE', #8945, #9988, #4878, .T. ) ;
#4968=CYLINDRICAL_SURFACE ( 'NONE', #2161, 5.499999999999986677 ) ;
#4970=DIRECTION ( 'NONE',  ( 0.6368676505102708330, 0.000000000000000000, 0.7709731485165535192 ) ) ;
#4979=ORIENTED_EDGE ( 'NONE', *, *, #6793, .T. ) ;
#4991=PRESENTATION_STYLE_ASSIGNMENT (( #935 ) ) ;
#4996=EDGE_CURVE ( 'NONE', #6924, #11433, #6594, .T. ) ;
#4998=ORIENTED_EDGE ( 'NONE', *, *, #1303, .F. ) ;
#5002=DIRECTION ( 'NONE',  ( -0.000000000000000000, -1.000000000000000000, 0.000000000000000000 ) ) ;
#5009=EDGE_CURVE ( 'NONE', #10885, #2640, #3164, .T. ) ;
#5014=ORIENTED_EDGE ( 'NONE', *, *, #5923, .F. ) ;
#5017=CARTESIAN_POINT ( 'NONE',  ( -31.19222893191934531, -19.00000000000000000, 286.4438302234617595 ) ) ;
#5026=EDGE_LOOP ( 'NONE', ( #5195, #10986, #715, #10684 ) ) ;
#5032=LINE ( 'NONE', #7113, #6012 ) ;
#5033=CARTESIAN_POINT ( 'NONE',  ( -225.1241593668336236, -30.00000000000000000, 185.9653539489990521 ) ) ;
#5036=EDGE_LOOP ( 'NONE', ( #2046, #4743 ) ) ;
#5039=ORIENTED_EDGE ( 'NONE', *, *, #2487, .F. ) ;
#5049=( LENGTH_UNIT ( ) NAMED_UNIT ( * ) SI_UNIT ( .MILLI., .METRE. ) );
#5060=DIRECTION ( 'NONE',  ( -0.6368676505102698338, 0.000000000000000000, -0.7709731485165541853 ) ) ;
#5061=EDGE_CURVE ( 'NONE', #9111, #10034, #13021, .T. ) ;
#5069=ORIENTED_EDGE ( 'NONE', *, *, #3028, .F. ) ;
#5086=ADVANCED_FACE ( 'NONE', ( #4888 ), #8024, .F. ) ;
#5094=CARTESIAN_POINT ( 'NONE',  ( 131.7449682071765835, -18.00000000000000000, -261.2053404739389180 ) ) ;
#5095=EDGE_CURVE ( 'NONE', #5893, #10423, #12155, .T. ) ;
#5098=CARTESIAN_POINT ( 'NONE',  ( 220.9845196385168435, -30.00000000000000000, -190.9766794143566528 ) ) ;
#5104=EDGE_LOOP ( 'NONE', ( #4194, #11843 ) ) ;
#5114=DIRECTION ( 'NONE',  ( 0.6368676505102695007, 0.000000000000000000, 0.7709731485165545184 ) ) ;
#5121=CARTESIAN_POINT ( 'NONE',  ( -23.54981712579611042, -18.00000000000000000, 295.6955080056604288 ) ) ;
#5124=VECTOR ( 'NONE', #3509, 1000.000000000000000 ) ;
#5133=CIRCLE ( 'NONE', #2785, 305.0000000000000000 ) ;
#5134=DIRECTION ( 'NONE',  ( 0.6368676505102706109, 0.000000000000000000, 0.7709731485165535192 ) ) ;
#5140=CONICAL_SURFACE ( 'NONE', #2792, 6.500000000000005329, 0.7853981633974518317 ) ;
#5145=DIRECTION ( 'NONE',  ( 0.6368676505102689456, 0.000000000000000000, 0.7709731485165549625 ) ) ;
#5148=LINE ( 'NONE', #12033, #11769 ) ;
#5152=ORIENTED_EDGE ( 'NONE', *, *, #10380, .T. ) ;
#5156=EDGE_CURVE ( 'NONE', #11433, #11239, #7854, .T. ) ;
#5160=AXIS2_PLACEMENT_3D ( 'NONE', #2435, #571, #318 ) ;
#5163=CARTESIAN_POINT ( 'NONE',  ( 286.5445428119865596, -18.00000000000000000, 22.67813138875427370 ) ) ;
#5164=DIRECTION ( 'NONE',  ( 0.000000000000000000, 1.000000000000000000, 0.000000000000000000 ) ) ;
#5166=DIRECTION ( 'NONE',  ( -0.000000000000000000, -1.000000000000000000, 0.000000000000000000 ) ) ;
#5169=EDGE_LOOP ( 'NONE', ( #3120, #10604, #6664, #10049 ) ) ;
#5173=EDGE_CURVE ( 'NONE', #3688, #3038, #9759, .T. ) ;
#5179=EDGE_CURVE ( 'NONE', #7165, #10853, #4950, .T. ) ;
#5189=AXIS2_PLACEMENT_3D ( 'NONE', #1274, #12473, #3324 ) ;
#5192=DIRECTION ( 'NONE',  ( -0.6368676505102737195, 0.000000000000000000, -0.7709731485165509657 ) ) ;
#5195=ORIENTED_EDGE ( 'NONE', *, *, #708, .F. ) ;
#5201=AXIS2_PLACEMENT_3D ( 'NONE', #4636, #3517, #12779 ) ;
#5210=CIRCLE ( 'NONE', #125, 5.100000000000017408 ) ;
#5214=VERTEX_POINT ( 'NONE', #5017 ) ;
#5215=FACE_OUTER_BOUND ( 'NONE', #8257, .T. ) ;
#5216=LINE ( 'NONE', #9290, #4858 ) ;
#5219=CARTESIAN_POINT ( 'NONE',  ( 159.3442861576696998, -29.00000000000000000, 192.8974817588416784 ) ) ;
#5221=CIRCLE ( 'NONE', #6935, 6.500000000000005329 ) ;
#5225=EDGE_CURVE ( 'NONE', #1921, #8685, #10146, .T. ) ;
#5227=DIRECTION ( 'NONE',  ( -0.4503334343941563511, -0.7071067811865480168, -0.5451603414287977678 ) ) ;
#5228=ORIENTED_EDGE ( 'NONE', *, *, #7989, .F. ) ;
#5230=AXIS2_PLACEMENT_3D ( 'NONE', #11414, #10337, #410 ) ;
#5233=CARTESIAN_POINT ( 'NONE',  ( 159.9811538081799540, 20.00000000000000000, 193.6684549073582673 ) ) ;
#5235=FACE_OUTER_BOUND ( 'NONE', #7847, .T. ) ;
#5239=DIRECTION ( 'NONE',  ( 0.6368676505102700558, 0.000000000000000000, 0.7709731485165541853 ) ) ;
#5240=DIRECTION ( 'NONE',  ( 0.6368676505102716101, 0.000000000000000000, 0.7709731485165527420 ) ) ;
#5260=EDGE_CURVE ( 'NONE', #11029, #9991, #2945, .T. ) ;
#5262=ORIENTED_EDGE ( 'NONE', *, *, #6118, .F. ) ;
#5271=DIRECTION ( 'NONE',  ( 0.6368676505102698338, 0.000000000000000000, 0.7709731485165541853 ) ) ;
#5275=ORIENTED_EDGE ( 'NONE', *, *, #9525, .F. ) ;
#5279=ORIENTED_EDGE ( 'NONE', *, *, #92, .F. ) ;
#5281=CARTESIAN_POINT ( 'NONE',  ( -27.68945685411286561, -19.00000000000000000, 290.6841825403027997 ) ) ;
#5287=EDGE_LOOP ( 'NONE', ( #3631, #12717, #9932, #8376 ) ) ;
#5295=ORIENTED_EDGE ( 'NONE', *, *, #1933, .F. ) ;
#5296=VECTOR ( 'NONE', #3953, 999.9999999999998863 ) ;
#5298=LINE ( 'NONE', #2493, #927 ) ;
#5300=DIRECTION ( 'NONE',  ( -0.000000000000000000, -1.000000000000000000, 0.000000000000000000 ) ) ;
#5304=VECTOR ( 'NONE', #7374, 1000.000000000000000 ) ;
#5307=CARTESIAN_POINT ( 'NONE',  ( 139.1326329530957082, -28.60000000000000142, -252.2620519511468729 ) ) ;
#5309=AXIS2_PLACEMENT_3D ( 'NONE', #4145, #11082, #4006 ) ;
#5310=ORIENTED_EDGE ( 'NONE', *, *, #3748, .T. ) ;
#5312=ORIENTED_EDGE ( 'NONE', *, *, #2991, .F. ) ;
#5315=AXIS2_PLACEMENT_3D ( 'NONE', #1238, #5300, #4297 ) ;
#5317=ORIENTED_EDGE ( 'NONE', *, *, #4463, .T. ) ;
#5327=ADVANCED_FACE ( 'NONE', ( #5215 ), #4150, .F. ) ;
#5328=EDGE_CURVE ( 'NONE', #9350, #6648, #12482, .T. ) ;
#5338=DIRECTION ( 'NONE',  ( 0.000000000000000000, 1.000000000000000000, 0.000000000000000000 ) ) ;
#5343=DIRECTION ( 'NONE',  ( 0.4503334343941555740, 0.7071067811865490160, 0.5451603414287971017 ) ) ;
#5352=CARTESIAN_POINT ( 'NONE',  ( -290.6841825403030839, -30.00000000000000000, -27.68945685411394919 ) ) ;
#5360=CARTESIAN_POINT ( 'NONE',  ( 225.1241593668336236, -29.00000000000000000, -185.9653539489990521 ) ) ;
#5364=CARTESIAN_POINT ( 'NONE',  ( -229.2637990951503753, -30.00000000000000000, 180.9540284836414514 ) ) ;
#5368=DIRECTION ( 'NONE',  ( -0.000000000000000000, -1.000000000000000000, 0.000000000000000000 ) ) ;
#5370=CARTESIAN_POINT ( 'NONE',  ( -0.000000000000000000, -30.00000000000000000, 0.000000000000000000 ) ) ;
#5374=CARTESIAN_POINT ( 'NONE',  ( 153.9282213272189495, -30.00000000000000000, 245.7765299597151341 ) ) ;
#5378=CARTESIAN_POINT ( 'NONE',  ( 135.8846079354933352, -19.40000000000000213, -256.1940150085812888 ) ) ;
#5380=EDGE_LOOP ( 'NONE', ( #5856, #10846, #2347, #11635 ) ) ;
#5382=CARTESIAN_POINT ( 'NONE',  ( -225.1241593668336236, -19.00000000000000000, 185.9653539489990521 ) ) ;
#5384=EDGE_CURVE ( 'NONE', #9508, #7035, #8504, .T. ) ;
#5391=AXIS2_PLACEMENT_3D ( 'NONE', #8222, #12145, #5134 ) ;
#5393=AXIS2_PLACEMENT_3D ( 'NONE', #833, #4690, #9960 ) ;
#5395=DIRECTION ( 'NONE',  ( 0.7709731485165535192, 0.000000000000000000, -0.6368676505102707219 ) ) ;
#5400=EDGE_LOOP ( 'NONE', ( #8773, #4162 ) ) ;
#5402=DIRECTION ( 'NONE',  ( -0.000000000000000000, -1.000000000000000000, 0.000000000000000000 ) ) ;
#5403=FACE_OUTER_BOUND ( 'NONE', #6353, .T. ) ;
#5405=DIRECTION ( 'NONE',  ( 0.6368676505102716101, 0.000000000000000000, 0.7709731485165527420 ) ) ;
#5406=ADVANCED_FACE ( 'NONE', ( #4084 ), #6297, .F. ) ;
#5411=CIRCLE ( 'NONE', #4760, 250.7000000000000171 ) ;
#5418=EDGE_LOOP ( 'NONE', ( #577, #1027, #1779, #12310 ) ) ;
#5422=AXIS2_PLACEMENT_3D ( 'NONE', #538, #4585, #8729 ) ;
#5425=CARTESIAN_POINT ( 'NONE',  ( -225.1241593668336236, -30.00000000000000000, 185.9653539489990521 ) ) ;
#5432=EDGE_CURVE ( 'NONE', #2079, #1416, #11217, .T. ) ;
#5435=ORIENTED_EDGE ( 'NONE', *, *, #708, .T. ) ;
#5450=CARTESIAN_POINT ( 'NONE',  ( -31.82909658242962792, -30.00000000000000000, 285.6728570749452274 ) ) ;
#5461=ORIENTED_EDGE ( 'NONE', *, *, #4667, .T. ) ;
#5463=DIRECTION ( 'NONE',  ( -0.000000000000000000, -1.000000000000000000, 0.000000000000000000 ) ) ;
#5464=DIRECTION ( 'NONE',  ( 0.6368676505102696117, 0.000000000000000000, 0.7709731485165545184 ) ) ;
#5465=CARTESIAN_POINT ( 'NONE',  ( 193.6077657551222444, -18.00000000000000000, 234.3758371490322361 ) ) ;
#5468=EDGE_CURVE ( 'NONE', #10757, #8455, #6784, .T. ) ;
#5477=ADVANCED_FACE ( 'NONE', ( #11556 ), #1029, .T. ) ;
#5478=CARTESIAN_POINT ( 'NONE',  ( -228.6269314446401211, -29.00000000000000000, 181.7250016321579835 ) ) ;
#5479=DIRECTION ( 'NONE',  ( 0.000000000000000000, -1.000000000000000000, 0.000000000000000000 ) ) ;
#5481=AXIS2_PLACEMENT_3D ( 'NONE', #1662, #12925, #11808 ) ;
#5491=ORIENTED_EDGE ( 'NONE', *, *, #9803, .T. ) ;
#5495=DIRECTION ( 'NONE',  ( 0.6368676505102716101, 0.000000000000000000, 0.7709731485165527420 ) ) ;
#5508=VERTEX_POINT ( 'NONE', #5478 ) ;
#5514=CYLINDRICAL_SURFACE ( 'NONE', #12560, 5.100000000000003197 ) ;
#5516=FACE_OUTER_BOUND ( 'NONE', #5889, .T. ) ;
#5524=CONICAL_SURFACE ( 'NONE', #5948, 5.500000000000015099, 0.7853981633974461696 ) ;
#5526=VERTEX_POINT ( 'NONE', #5544 ) ;
#5529=DIRECTION ( 'NONE',  ( 0.6368676505102707219, 0.000000000000000000, 0.7709731485165535192 ) ) ;
#5530=LINE ( 'NONE', #9471, #10429 ) ;
#5540=ADVANCED_FACE ( 'NONE', ( #8552 ), #7485, .F. ) ;
#5544=CARTESIAN_POINT ( 'NONE',  ( 228.6269314446401211, -19.00000000000000000, -181.7250016321579835 ) ) ;
#5557=ORIENTED_EDGE ( 'NONE', *, *, #7831, .F. ) ;
#5560=VECTOR ( 'NONE', #12171, 1000.000000000000000 ) ;
#5576=DIRECTION ( 'NONE',  ( -0.000000000000000000, -1.000000000000000000, 0.000000000000000000 ) ) ;
#5577=DIRECTION ( 'NONE',  ( 0.6368676505102707219, 0.000000000000000000, 0.7709731485165535192 ) ) ;
#5578=DIRECTION ( 'NONE',  ( -0.000000000000000000, -1.000000000000000000, 0.000000000000000000 ) ) ;
#5579=AXIS2_PLACEMENT_3D ( 'NONE', #11619, #4465, #6488 ) ;
#5583=EDGE_CURVE ( 'NONE', #9146, #4062, #4469, .T. ) ;
#5597=VECTOR ( 'NONE', #1772, 1000.000000000000000 ) ;
#5605=CONICAL_SURFACE ( 'NONE', #9014, 5.100000000000003197, 0.7853981633974503884 ) ;
#5610=ORIENTED_EDGE ( 'NONE', *, *, #8812, .T. ) ;
#5611=VERTEX_POINT ( 'NONE', #3670 ) ;
#5620=ADVANCED_FACE ( 'NONE', ( #10606 ), #1457, .F. ) ;
#5624=ORIENTED_EDGE ( 'NONE', *, *, #12015, .F. ) ;
#5625=CARTESIAN_POINT ( 'NONE',  ( -27.68945685411286561, -18.00000000000000000, 290.6841825403027997 ) ) ;
#5626=ORIENTED_EDGE ( 'NONE', *, *, #5009, .T. ) ;
#5631=DIRECTION ( 'NONE',  ( -0.4503334343941441942, 0.7071067811865670016, -0.5451603414287832239 ) ) ;
#5632=LINE ( 'NONE', #11963, #3237 ) ;
#5647=DIRECTION ( 'NONE',  ( -0.000000000000000000, -1.000000000000000000, 0.000000000000000000 ) ) ;
#5649=DIRECTION ( 'NONE',  ( 0.6368676505102716101, 0.000000000000000000, 0.7709731485165527420 ) ) ;
#5650=AXIS2_PLACEMENT_3D ( 'NONE', #3575, #4634, #7647 ) ;
#5658=ORIENTED_EDGE ( 'NONE', *, *, #2487, .T. ) ;
#5662=DIRECTION ( 'NONE',  ( -0.000000000000000000, -1.000000000000000000, 0.000000000000000000 ) ) ;
#5666=EDGE_CURVE ( 'NONE', #9649, #779, #4861, .T. ) ;
#5671=CARTESIAN_POINT ( 'NONE',  ( 225.1241593668336236, -30.00000000000000000, -185.9653539489990521 ) ) ;
#5672=CARTESIAN_POINT ( 'NONE',  ( 27.68945685411497593, -19.00000000000000000, -290.6841825403026291 ) ) ;
#5674=ORIENTED_EDGE ( 'NONE', *, *, #1828, .F. ) ;
#5676=DIRECTION ( 'NONE',  ( -0.000000000000000000, -1.000000000000000000, 0.000000000000000000 ) ) ;
#5677=EDGE_CURVE ( 'NONE', #11199, #9111, #6357, .T. ) ;
#5681=DIRECTION ( 'NONE',  ( -0.000000000000000000, -1.000000000000000000, 0.000000000000000000 ) ) ;
#5684=CARTESIAN_POINT ( 'NONE',  ( 31.82909658243172757, -18.00000000000000000, -285.6728570749450569 ) ) ;
#5687=CARTESIAN_POINT ( 'NONE',  ( 27.68945685411497593, -29.00000000000000000, -290.6841825403026291 ) ) ;
#5693=LINE ( 'NONE', #7760, #7944 ) ;
#5701=FACE_OUTER_BOUND ( 'NONE', #5380, .T. ) ;
#5704=ORIENTED_EDGE ( 'NONE', *, *, #12058, .T. ) ;
#5708=DIRECTION ( 'NONE',  ( 0.6368676505102689456, 0.000000000000000000, 0.7709731485165549625 ) ) ;
#5709=CARTESIAN_POINT ( 'NONE',  ( 194.2446334056325554, -19.00000000000000000, 235.1468102975488250 ) ) ;
#5710=DIRECTION ( 'NONE',  ( -0.000000000000000000, -1.000000000000000000, 0.000000000000000000 ) ) ;
#5715=EDGE_LOOP ( 'NONE', ( #11385, #12282, #2374, #3649 ) ) ;
#5717=ORIENTED_EDGE ( 'NONE', *, *, #12845, .F. ) ;
#5718=CIRCLE ( 'NONE', #1520, 6.500000000000005329 ) ;
#5722=AXIS2_PLACEMENT_3D ( 'NONE', #957, #2872, #9024 ) ;
#5723=EDGE_LOOP ( 'NONE', ( #6855, #11215, #9299, #7037 ) ) ;
#5742=ORIENTED_EDGE ( 'NONE', *, *, #8425, .F. ) ;
#5752=DIRECTION ( 'NONE',  ( -0.000000000000000000, -1.000000000000000000, 0.000000000000000000 ) ) ;
#5755=ORIENTED_EDGE ( 'NONE', *, *, #2712, .F. ) ;
#5759=ORIENTED_EDGE ( 'NONE', *, *, #4966, .F. ) ;
#5760=EDGE_CURVE ( 'NONE', #5526, #9991, #12875, .T. ) ;
#5762=VERTEX_POINT ( 'NONE', #11001 ) ;
#5769=EDGE_LOOP ( 'NONE', ( #10987, #7450, #12514, #4175 ) ) ;
#5770=DIRECTION ( 'NONE',  ( -0.4503334343941691187, -0.7071067811865280328, -0.5451603414288131999 ) ) ;
#5773=EDGE_LOOP ( 'NONE', ( #222, #7318 ) ) ;
#5779=DIRECTION ( 'NONE',  ( 0.6368676505102708330, 0.000000000000000000, 0.7709731485165535192 ) ) ;
#5793=ORIENTED_EDGE ( 'NONE', *, *, #8650, .T. ) ;
#5797=LINE ( 'NONE', #4714, #10621 ) ;
#5798=CIRCLE ( 'NONE', #688, 250.1999999999999602 ) ;
#5814=DIRECTION ( 'NONE',  ( 0.000000000000000000, 1.000000000000000000, 0.000000000000000000 ) ) ;
#5816=EDGE_CURVE ( 'NONE', #7165, #11682, #3726, .T. ) ;
#5819=CARTESIAN_POINT ( 'NONE',  ( -290.6841825403030839, -19.00000000000000000, -27.68945685411394919 ) ) ;
#5824=DIRECTION ( 'NONE',  ( 0.4503334343941574613, 0.7071067811865460184, 0.5451603414287994331 ) ) ;
#5825=VERTEX_POINT ( 'NONE', #943 ) ;
#5830=CONICAL_SURFACE ( 'NONE', #3476, 5.500000000000007994, 0.7853981633974461696 ) ;
#5833=ORIENTED_EDGE ( 'NONE', *, *, #3491, .F. ) ;
#5834=AXIS2_PLACEMENT_3D ( 'NONE', #539, #7469, #11607 ) ;
#5837=EDGE_CURVE ( 'NONE', #5907, #3975, #4687, .T. ) ;
#5850=LINE ( 'NONE', #10102, #31 ) ;
#5852=CARTESIAN_POINT ( 'NONE',  ( 132.6365829178909621, -28.60000000000000142, -260.1259780660157048 ) ) ;
#5856=ORIENTED_EDGE ( 'NONE', *, *, #3871, .T. ) ;
#5857=DIRECTION ( 'NONE',  ( 0.6368676505102707219, 0.000000000000000000, 0.7709731485165536302 ) ) ;
#5861=VERTEX_POINT ( 'NONE', #3788 ) ;
#5862=FACE_OUTER_BOUND ( 'NONE', #2877, .T. ) ;
#5863=EDGE_LOOP ( 'NONE', ( #5624, #8992, #1633, #6370 ) ) ;
#5866=DIRECTION ( 'NONE',  ( 0.6368676505102707219, 0.000000000000000000, 0.7709731485165536302 ) ) ;
#5878=ORIENTED_EDGE ( 'NONE', *, *, #8334, .T. ) ;
#5880=AXIS2_PLACEMENT_3D ( 'NONE', #877, #5002, #1941 ) ;
#5882=DIRECTION ( 'NONE',  ( -0.6368676505102700558, 0.000000000000000000, -0.7709731485165541853 ) ) ;
#5886=CYLINDRICAL_SURFACE ( 'NONE', #2403, 5.500000000000007994 ) ;
#5888=CARTESIAN_POINT ( 'NONE',  ( 0.000000000000000000, 0.000000000000000000, 0.000000000000000000 ) ) ;
#5889=EDGE_LOOP ( 'NONE', ( #4824, #7154, #8687, #9055 ) ) ;
#5893=VERTEX_POINT ( 'NONE', #12199 ) ;
#5895=ORIENTED_EDGE ( 'NONE', *, *, #2638, .T. ) ;
#5904=ORIENTED_EDGE ( 'NONE', *, *, #9245, .T. ) ;
#5907=VERTEX_POINT ( 'NONE', #3051 ) ;
#5922=VERTEX_POINT ( 'NONE', #4856 ) ;
#5923=EDGE_CURVE ( 'NONE', #12436, #9350, #5210, .T. ) ;
#5926=EDGE_LOOP ( 'NONE', ( #3918, #660, #9217, #6011 ) ) ;
#5929=FACE_OUTER_BOUND ( 'NONE', #10813, .T. ) ;
#5935=MANIFOLD_SOLID_BREP ( 'NONE', #4530 ) ;
#5938=AXIS2_PLACEMENT_3D ( 'NONE', #2378, #6453, #9383 ) ;
#5939=CARTESIAN_POINT ( 'NONE',  ( 27.68945685411497593, -19.00000000000000000, -290.6841825403026291 ) ) ;
#5946=EDGE_LOOP ( 'NONE', ( #7241, #1067, #3362, #6220 ) ) ;
#5948=AXIS2_PLACEMENT_3D ( 'NONE', #6396, #1516, #11655 ) ;
#5950=DIRECTION ( 'NONE',  ( -0.000000000000000000, -1.000000000000000000, 0.000000000000000000 ) ) ;
#5957=EDGE_CURVE ( 'NONE', #366, #2076, #2026, .T. ) ;
#5965=DIRECTION ( 'NONE',  ( -0.4503334343941582940, -0.7071067811865450192, -0.5451603414288000993 ) ) ;
#5969=CIRCLE ( 'NONE', #217, 5.499999999999986677 ) ;
#5971=CARTESIAN_POINT ( 'NONE',  ( 220.9845196385168435, -30.00000000000000000, -190.9766794143566528 ) ) ;
#5979=DIRECTION ( 'NONE',  ( 0.6368676505102695007, 0.000000000000000000, 0.7709731485165545184 ) ) ;
#5981=EDGE_CURVE ( 'NONE', #4180, #2618, #7328, .T. ) ;
#5983=EDGE_CURVE ( 'NONE', #9116, #12435, #10543, .T. ) ;
#5984=DIRECTION ( 'NONE',  ( 0.4503334343941574613, 0.7071067811865460184, 0.5451603414287994331 ) ) ;
#5996=AXIS2_PLACEMENT_3D ( 'NONE', #12243, #3966, #2037 ) ;
#6003=EDGE_CURVE ( 'NONE', #7702, #1100, #4788, .T. ) ;
#6007=CARTESIAN_POINT ( 'NONE',  ( -221.6213872890270977, -19.00000000000000000, 190.2057062658400923 ) ) ;
#6011=ORIENTED_EDGE ( 'NONE', *, *, #8650, .F. ) ;
#6012=VECTOR ( 'NONE', #118, 1000.000000000000000 ) ;
#6013=DIRECTION ( 'NONE',  ( -0.000000000000000000, -1.000000000000000000, 0.000000000000000000 ) ) ;
#6020=AXIS2_PLACEMENT_3D ( 'NONE', #7891, #6164, #1092 ) ;
#6031=CIRCLE ( 'NONE', #12626, 251.1999999999999886 ) ;
#6045=CARTESIAN_POINT ( 'NONE',  ( -159.3442861576697283, 0.000000000000000000, -192.8974817588416499 ) ) ;
#6047=CYLINDRICAL_SURFACE ( 'NONE', #626, 270.0000000000000000 ) ;
#6060=EDGE_CURVE ( 'NONE', #10237, #3272, #8594, .T. ) ;
#6061=AXIS2_PLACEMENT_3D ( 'NONE', #1240, #12502, #12636 ) ;
#6063=ORIENTED_EDGE ( 'NONE', *, *, #7034, .T. ) ;
#6066=FACE_OUTER_BOUND ( 'NONE', #5769, .T. ) ;
#6069=CIRCLE ( 'NONE', #1807, 260.1830065359559967 ) ;
#6077=ORIENTED_EDGE ( 'NONE', *, *, #6698, .F. ) ;
#6081=EDGE_CURVE ( 'NONE', #5508, #2601, #11404, .T. ) ;
#6088=AXIS2_PLACEMENT_3D ( 'NONE', #2698, #9702, #2579 ) ;
#6090=CARTESIAN_POINT ( 'NONE',  ( -0.000000000000000000, -22.00000000000000000, 0.000000000000000000 ) ) ;
#6101=ORIENTED_EDGE ( 'NONE', *, *, #10363, .T. ) ;
#6105=EDGE_LOOP ( 'NONE', ( #10960, #2110, #6434, #11286 ) ) ;
#6106=LINE ( 'NONE', #6045, #673 ) ;
#6107=CARTESIAN_POINT ( 'NONE',  ( 153.9282213272189495, -30.00000000000000000, 245.7765299597151341 ) ) ;
#6108=CARTESIAN_POINT ( 'NONE',  ( 161.8917567597108018, 0.000000000000000000, 195.9813743529078920 ) ) ;
#6111=DIRECTION ( 'NONE',  ( -0.000000000000000000, -1.000000000000000000, 0.000000000000000000 ) ) ;
#6113=ORIENTED_EDGE ( 'NONE', *, *, #4231, .F. ) ;
#6118=EDGE_CURVE ( 'NONE', #11136, #5861, #6595, .T. ) ;
#6119=EDGE_CURVE ( 'NONE', #6702, #1100, #4572, .T. ) ;
#6126=CIRCLE ( 'NONE', #12508, 250.1999999999999602 ) ;
#6140=CARTESIAN_POINT ( 'NONE',  ( 149.7885815989021694, -30.00000000000000000, 240.7652044943575333 ) ) ;
#6141=DIRECTION ( 'NONE',  ( -0.000000000000000000, -1.000000000000000000, 0.000000000000000000 ) ) ;
#6147=ADVANCED_FACE ( 'NONE', ( #12712 ), #4705, .F. ) ;
#6148=CARTESIAN_POINT ( 'NONE',  ( -287.1814104624966149, -19.00000000000000000, -23.44910453727290545 ) ) ;
#6153=DIRECTION ( 'NONE',  ( 0.000000000000000000, 1.000000000000000000, 0.000000000000000000 ) ) ;
#6160=AXIS2_PLACEMENT_3D ( 'NONE', #4117, #3041, #64 ) ;
#6163=ADVANCED_FACE ( 'NONE', ( #11724 ), #11189, .F. ) ;
#6164=DIRECTION ( 'NONE',  ( -0.000000000000000000, -1.000000000000000000, 0.000000000000000000 ) ) ;
#6168=AXIS2_PLACEMENT_3D ( 'NONE', #11308, #9104, #910 ) ;
#6170=DIRECTION ( 'NONE',  ( 0.4503334343941562956, -0.7071067811865480168, 0.5451603414287978788 ) ) ;
#6195=DIRECTION ( 'NONE',  ( -0.000000000000000000, -1.000000000000000000, 0.000000000000000000 ) ) ;
#6198=EDGE_CURVE ( 'NONE', #1725, #8820, #1187, .T. ) ;
#6199=EDGE_LOOP ( 'NONE', ( #5069, #9711, #8824, #5295 ) ) ;
#6212=DIRECTION ( 'NONE',  ( -0.000000000000000000, -1.000000000000000000, 0.000000000000000000 ) ) ;
#6220=ORIENTED_EDGE ( 'NONE', *, *, #12321, .F. ) ;
#6221=AXIS2_PLACEMENT_3D ( 'NONE', #12306, #7245, #2371 ) ;
#6222=CARTESIAN_POINT ( 'NONE',  ( -294.1869546181095529, -19.00000000000000000, -31.92980917095500359 ) ) ;
#6226=EDGE_CURVE ( 'NONE', #1949, #11299, #7064, .T. ) ;
#6231=CONICAL_SURFACE ( 'NONE', #2595, 6.500000000000000888, 0.7853981633974617127 ) ;
#6235=VECTOR ( 'NONE', #4071, 1000.000000000000000 ) ;
#6241=EDGE_LOOP ( 'NONE', ( #984, #890, #4401, #3334 ) ) ;
#6246=CARTESIAN_POINT ( 'NONE',  ( -0.000000000000000000, -25.00000000000000000, 0.000000000000000000 ) ) ;
#6256=AXIS2_PLACEMENT_3D ( 'NONE', #2462, #6409, #5464 ) ;
#6259=ORIENTED_EDGE ( 'NONE', *, *, #10275, .T. ) ;
#6261=DIRECTION ( 'NONE',  ( -0.000000000000000000, -1.000000000000000000, 0.000000000000000000 ) ) ;
#6268=CARTESIAN_POINT ( 'NONE',  ( 287.1814104624967854, -29.00000000000000000, 23.44910453727084132 ) ) ;
#6273=AXIS2_PLACEMENT_3D ( 'NONE', #1314, #2966, #5239 ) ;
#6281=FACE_BOUND ( 'NONE', #8725, .T. ) ;
#6282=CIRCLE ( 'NONE', #12874, 304.0000000000000000 ) ;
#6290=( GEOMETRIC_REPRESENTATION_CONTEXT ( 3 ) GLOBAL_UNCERTAINTY_ASSIGNED_CONTEXT ( ( #919 ) ) GLOBAL_UNIT_ASSIGNED_CONTEXT ( ( #5049, #9327, #2257 ) ) REPRESENTATION_CONTEXT ( 'NONE', 'WORKASPACE' ) );
#6296=ADVANCED_FACE ( 'NONE', ( #11237 ), #9062, .F. ) ;
#6297=CYLINDRICAL_SURFACE ( 'NONE', #9117, 5.499999999999986677 ) ;
#6304=ORIENTED_EDGE ( 'NONE', *, *, #4083, .T. ) ;
#6309=ORIENTED_EDGE ( 'NONE', *, *, #6858, .T. ) ;
#6310=AXIS2_PLACEMENT_3D ( 'NONE', #9081, #8017, #12076 ) ;
#6317=DIRECTION ( 'NONE',  ( 0.6368676505102707219, 0.000000000000000000, 0.7709731485165535192 ) ) ;
#6318=ADVANCED_FACE ( 'NONE', ( #3482 ), #3944, .T. ) ;
#6321=CARTESIAN_POINT ( 'NONE',  ( -0.000000000000000000, -3.061616997868385015E-14, 0.000000000000000000 ) ) ;
#6337=ORIENTED_EDGE ( 'NONE', *, *, #2863, .T. ) ;
#6346=DIRECTION ( 'NONE',  ( -0.7709731485165536302, 0.000000000000000000, 0.6368676505102706109 ) ) ;
#6353=EDGE_LOOP ( 'NONE', ( #2766, #11268, #12575, #9811 ) ) ;
#6355=CARTESIAN_POINT ( 'NONE',  ( 225.1241593668336236, -29.00000000000000000, -185.9653539489990521 ) ) ;
#6357=CIRCLE ( 'NONE', #12951, 5.500000000000015099 ) ;
#6361=DIRECTION ( 'NONE',  ( 0.6368676505102709440, 0.000000000000000000, 0.7709731485165532971 ) ) ;
#6365=ADVANCED_FACE ( 'NONE', ( #1619 ), #11882, .F. ) ;
#6366=EDGE_LOOP ( 'NONE', ( #4360, #3779, #6945, #12965 ) ) ;
#6367=AXIS2_PLACEMENT_3D ( 'NONE', #10373, #1247, #250 ) ;
#6370=ORIENTED_EDGE ( 'NONE', *, *, #512, .F. ) ;
#6371=VECTOR ( 'NONE', #435, 1000.000000000000000 ) ;
#6374=ORIENTED_EDGE ( 'NONE', *, *, #3862, .F. ) ;
#6375=CONICAL_SURFACE ( 'NONE', #5422, 5.499999999999986677, 0.7853981633974461696 ) ;
#6376=AXIS2_PLACEMENT_3D ( 'NONE', #2522, #4387, #3383 ) ;
#6380=DIRECTION ( 'NONE',  ( -0.000000000000000000, -1.000000000000000000, 0.000000000000000000 ) ) ;
#6388=AXIS2_PLACEMENT_3D ( 'NONE', #10631, #1499, #10504 ) ;
#6396=CARTESIAN_POINT ( 'NONE',  ( 185.9653539490014111, -19.00000000000000000, 225.1241593668316625 ) ) ;
#6397=DIRECTION ( 'NONE',  ( -0.000000000000000000, -1.000000000000000000, 0.000000000000000000 ) ) ;
#6404=DIRECTION ( 'NONE',  ( -0.6368676505102689456, 0.000000000000000000, -0.7709731485165549625 ) ) ;
#6405=ORIENTED_EDGE ( 'NONE', *, *, #11171, .F. ) ;
#6407=EDGE_CURVE ( 'NONE', #10097, #11992, #11825, .T. ) ;
#6409=DIRECTION ( 'NONE',  ( -0.000000000000000000, -1.000000000000000000, 0.000000000000000000 ) ) ;
#6428=DIRECTION ( 'NONE',  ( -0.000000000000000000, -1.000000000000000000, 0.000000000000000000 ) ) ;
#6434=ORIENTED_EDGE ( 'NONE', *, *, #4038, .F. ) ;
#6436=EDGE_LOOP ( 'NONE', ( #2700, #245, #873, #6617 ) ) ;
#6437=DIRECTION ( 'NONE',  ( 0.000000000000000000, 1.000000000000000000, 0.000000000000000000 ) ) ;
#6438=ORIENTED_EDGE ( 'NONE', *, *, #8205, .T. ) ;
#6440=CONICAL_SURFACE ( 'NONE', #6221, 6.500000000000005329, 0.7853981633974547183 ) ;
#6443=DIRECTION ( 'NONE',  ( -0.000000000000000000, -1.000000000000000000, 0.000000000000000000 ) ) ;
#6446=DIRECTION ( 'NONE',  ( 0.7709731485165535192, -0.000000000000000000, -0.6368676505102707219 ) ) ;
#6447=CIRCLE ( 'NONE', #3018, 5.100000000000017408 ) ;
#6450=AXIS2_PLACEMENT_3D ( 'NONE', #6623, #3809, #558 ) ;
#6453=DIRECTION ( 'NONE',  ( -0.000000000000000000, -1.000000000000000000, 0.000000000000000000 ) ) ;
#6458=EDGE_CURVE ( 'NONE', #12436, #2275, #10879, .T. ) ;
#6463=DIRECTION ( 'NONE',  ( -0.6368676505102706109, 0.000000000000000000, -0.7709731485165535192 ) ) ;
#6464=AXIS2_PLACEMENT_3D ( 'NONE', #11089, #4015, #12288 ) ;
#6467=ADVANCED_FACE ( 'NONE', ( #10950 ), #1820, .F. ) ;
#6474=ORIENTED_EDGE ( 'NONE', *, *, #7766, .F. ) ;
#6483=VECTOR ( 'NONE', #5463, 1000.000000000000000 ) ;
#6484=ADVANCED_FACE ( 'NONE', ( #12686 ), #12682, .F. ) ;
#6486=EDGE_CURVE ( 'NONE', #4412, #2618, #8644, .T. ) ;
#6488=DIRECTION ( 'NONE',  ( -0.6368676505102707219, 0.000000000000000000, -0.7709731485165536302 ) ) ;
#6491=VECTOR ( 'NONE', #8187, 1000.000000000000000 ) ;
#6494=CARTESIAN_POINT ( 'NONE',  ( 185.9653539490014111, -18.00000000000000000, 225.1241593668316625 ) ) ;
#6497=DIRECTION ( 'NONE',  ( -0.000000000000000000, -1.000000000000000000, 0.000000000000000000 ) ) ;
#6499=CARTESIAN_POINT ( 'NONE',  ( -185.9653539489998195, -30.00000000000000000, -225.1241593668329699 ) ) ;
#6501=AXIS2_PLACEMENT_3D ( 'NONE', #7266, #5395, #9268 ) ;
#6505=EDGE_LOOP ( 'NONE', ( #11918, #10951, #235, #6374 ) ) ;
#6506=CARTESIAN_POINT ( 'NONE',  ( 0.000000000000000000, 0.000000000000000000, 0.000000000000000000 ) ) ;
#6509=AXIS2_PLACEMENT_3D ( 'NONE', #1327, #1200, #8400 ) ;
#6512=DIRECTION ( 'NONE',  ( 0.6368676505102716101, 0.000000000000000000, 0.7709731485165527420 ) ) ;
#6517=ORIENTED_EDGE ( 'NONE', *, *, #3005, .T. ) ;
#6518=FACE_OUTER_BOUND ( 'NONE', #6105, .T. ) ;
#6519=AXIS2_PLACEMENT_3D ( 'NONE', #3513, #9644, #7585 ) ;
#6522=DIRECTION ( 'NONE',  ( -0.000000000000000000, -1.000000000000000000, 0.000000000000000000 ) ) ;
#6529=EDGE_CURVE ( 'NONE', #1416, #10031, #557, .T. ) ;
#6546=LINE ( 'NONE', #1280, #10338 ) ;
#6555=EDGE_CURVE ( 'NONE', #5526, #8820, #6546, .T. ) ;
#6556=EDGE_CURVE ( 'NONE', #5893, #11136, #4583, .T. ) ;
#6564=ORIENTED_EDGE ( 'NONE', *, *, #2923, .F. ) ;
#6567=CARTESIAN_POINT ( 'NONE',  ( -161.8917567597108587, -25.00000000000000000, -195.9813743529078636 ) ) ;
#6568=EDGE_LOOP ( 'NONE', ( #6405, #4550, #8840, #7917 ) ) ;
#6569=VERTEX_POINT ( 'NONE', #282 ) ;
#6570=DIRECTION ( 'NONE',  ( -0.4503334343941595708, -0.7071067811865430208, -0.5451603414288016536 ) ) ;
#6578=AXIS2_PLACEMENT_3D ( 'NONE', #12678, #3538, #11683 ) ;
#6585=DIRECTION ( 'NONE',  ( -0.6368676505102707219, 0.000000000000000000, -0.7709731485165535192 ) ) ;
#6589=FACE_OUTER_BOUND ( 'NONE', #8502, .T. ) ;
#6591=CARTESIAN_POINT ( 'NONE',  ( -0.000000000000000000, -9.830508068730530624, 0.000000000000000000 ) ) ;
#6592=CIRCLE ( 'NONE', #9165, 254.1999999999999886 ) ;
#6594=CIRCLE ( 'NONE', #6160, 2.000000000000000444 ) ;
#6595=LINE ( 'NONE', #9772, #6934 ) ;
#6597=CARTESIAN_POINT ( 'NONE',  ( 159.3442861576696714, 11.79660968244693997, 192.8974817588417068 ) ) ;
#6604=DIRECTION ( 'NONE',  ( -0.6368676505102707219, 0.000000000000000000, -0.7709731485165535192 ) ) ;
#6608=CARTESIAN_POINT ( 'NONE',  ( -181.8257142206830679, -18.00000000000000000, -220.1128339014753692 ) ) ;
#6610=DIRECTION ( 'NONE',  ( 0.6368676505102696117, 0.000000000000000000, 0.7709731485165545184 ) ) ;
#6614=DIRECTION ( 'NONE',  ( -0.000000000000000000, -1.000000000000000000, 0.000000000000000000 ) ) ;
#6617=ORIENTED_EDGE ( 'NONE', *, *, #6973, .T. ) ;
#6620=FACE_BOUND ( 'NONE', #1984, .T. ) ;
#6621=ADVANCED_FACE ( 'NONE', ( #9281 ), #7558, .T. ) ;
#6623=CARTESIAN_POINT ( 'NONE',  ( -289.8128292627096130, -30.00000000000000000, 10.41748504886635907 ) ) ;
#6626=DIRECTION ( 'NONE',  ( 0.6368676505102689456, 0.000000000000000000, 0.7709731485165549625 ) ) ;
#6631=ORIENTED_EDGE ( 'NONE', *, *, #3577, .T. ) ;
#6633=DIRECTION ( 'NONE',  ( 0.6368676505102709440, 0.000000000000000000, 0.7709731485165532971 ) ) ;
#6634=ORIENTED_EDGE ( 'NONE', *, *, #11991, .F. ) ;
#6645=ORIENTED_EDGE ( 'NONE', *, *, #2556, .T. ) ;
#6647=EDGE_CURVE ( 'NONE', #1953, #1244, #9256, .T. ) ;
#6648=VERTEX_POINT ( 'NONE', #12537 ) ;
#6649=EDGE_CURVE ( 'NONE', #10082, #10483, #9670, .T. ) ;
#6657=DIRECTION ( 'NONE',  ( 0.6368676505102696117, 0.000000000000000000, 0.7709731485165545184 ) ) ;
#6660=CARTESIAN_POINT ( 'NONE',  ( 0.000000000000000000, 11.79660968244693997, 0.000000000000000000 ) ) ;
#6661=DIRECTION ( 'NONE',  ( -0.000000000000000000, -1.000000000000000000, 0.000000000000000000 ) ) ;
#6664=ORIENTED_EDGE ( 'NONE', *, *, #11893, .T. ) ;
#6666=ORIENTED_EDGE ( 'NONE', *, *, #2863, .F. ) ;
#6675=CARTESIAN_POINT ( 'NONE',  ( -286.5648042451072115, -19.40000000000000213, 14.34944810630078393 ) ) ;
#6679=VECTOR ( 'NONE', #4295, 1000.000000000000000 ) ;
#6681=TOROIDAL_SURFACE ( 'NONE', #2821, 250.0000000000000000, 10.00000000000000000 ) ;
#6687=ORIENTED_EDGE ( 'NONE', *, *, #986, .F. ) ;
#6690=DIRECTION ( 'NONE',  ( -0.000000000000000000, -1.000000000000000000, 0.000000000000000000 ) ) ;
#6693=FACE_OUTER_BOUND ( 'NONE', #8944, .T. ) ;
#6698=EDGE_CURVE ( 'NONE', #2361, #9366, #9040, .T. ) ;
#6701=LINE ( 'NONE', #10687, #2944 ) ;
#6702=VERTEX_POINT ( 'NONE', #3791 ) ;
#6711=CARTESIAN_POINT ( 'NONE',  ( 0.000000000000000000, 0.000000000000000000, 0.000000000000000000 ) ) ;
#6721=FACE_OUTER_BOUND ( 'NONE', #3912, .T. ) ;
#6725=EDGE_CURVE ( 'NONE', #4180, #9382, #112, .T. ) ;
#6738=CARTESIAN_POINT ( 'NONE',  ( -294.1869546181095529, -19.00000000000000000, -31.92980917095498938 ) ) ;
#6749=FACE_OUTER_BOUND ( 'NONE', #11351, .T. ) ;
#6750=CARTESIAN_POINT ( 'NONE',  ( -0.000000000000000000, -19.00000000000000000, 0.000000000000000000 ) ) ;
#6753=DIRECTION ( 'NONE',  ( -0.000000000000000000, -1.000000000000000000, 0.000000000000000000 ) ) ;
#6770=LINE ( 'NONE', #10760, #10848 ) ;
#6771=ADVANCED_FACE ( 'NONE', ( #9196 ), #11129, .F. ) ;
#6778=ORIENTED_EDGE ( 'NONE', *, *, #5837, .T. ) ;
#6782=DIRECTION ( 'NONE',  ( -0.6368676505102700558, 0.000000000000000000, -0.7709731485165541853 ) ) ;
#6784=CIRCLE ( 'NONE', #10817, 5.100000000000003197 ) ;
#6789=VERTEX_POINT ( 'NONE', #1935 ) ;
#6793=EDGE_CURVE ( 'NONE', #941, #1921, #6282, .T. ) ;
#6795=EDGE_CURVE ( 'NONE', #8227, #10637, #3860, .T. ) ;
#6796=ORIENTED_EDGE ( 'NONE', *, *, #12176, .T. ) ;
#6797=AXIS2_PLACEMENT_3D ( 'NONE', #7184, #9056, #187 ) ;
#6808=CONICAL_SURFACE ( 'NONE', #8513, 5.500000000000015099, 0.7853981633974461696 ) ;
#6814=ORIENTED_EDGE ( 'NONE', *, *, #9012, .T. ) ;
#6815=VECTOR ( 'NONE', #2431, 1000.000000000000000 ) ;
#6817=CARTESIAN_POINT ( 'NONE',  ( -225.1241593668336236, -19.00000000000000000, 185.9653539489990521 ) ) ;
#6822=DIRECTION ( 'NONE',  ( 0.000000000000000000, 1.000000000000000000, 0.000000000000000000 ) ) ;
#6829=DIRECTION ( 'NONE',  ( 0.4503334343941441387, 0.7071067811865670016, 0.5451603414287832239 ) ) ;
#6836=ORIENTED_EDGE ( 'NONE', *, *, #4554, .F. ) ;
#6837=CARTESIAN_POINT ( 'NONE',  ( -0.000000000000000000, -21.50000000000000000, 0.000000000000000000 ) ) ;
#6840=ORIENTED_EDGE ( 'NONE', *, *, #535, .T. ) ;
#6843=DIRECTION ( 'NONE',  ( -0.000000000000000000, -1.000000000000000000, 0.000000000000000000 ) ) ;
#6845=DIRECTION ( 'NONE',  ( -0.000000000000000000, -1.000000000000000000, 0.000000000000000000 ) ) ;
#6855=ORIENTED_EDGE ( 'NONE', *, *, #1252, .T. ) ;
#6858=EDGE_CURVE ( 'NONE', #10530, #2838, #3279, .T. ) ;
#6859=EDGE_CURVE ( 'NONE', #7354, #2094, #11389, .T. ) ;
#6865=DIRECTION ( 'NONE',  ( 0.000000000000000000, 1.000000000000000000, 0.000000000000000000 ) ) ;
#6874=CIRCLE ( 'NONE', #2801, 6.500000000000026645 ) ;
#6888=CIRCLE ( 'NONE', #8387, 6.500000000000005329 ) ;
#6889=CIRCLE ( 'NONE', #12001, 2.000000000000000444 ) ;
#6891=CONICAL_SURFACE ( 'NONE', #1781, 5.100000000000003197, 0.7853981633974461696 ) ;
#6895=FACE_OUTER_BOUND ( 'NONE', #3866, .T. ) ;
#6903=EDGE_CURVE ( 'NONE', #3038, #3688, #6069, .T. ) ;
#6904=CARTESIAN_POINT ( 'NONE',  ( 189.4681260268079086, -19.00000000000000000, 229.3645116836727311 ) ) ;
#6924=VERTEX_POINT ( 'NONE', #4258 ) ;
#6926=ORIENTED_EDGE ( 'NONE', *, *, #3786, .T. ) ;
#6933=CARTESIAN_POINT ( 'NONE',  ( -31.19222893191935242, -19.00000000000000000, 286.4438302234617595 ) ) ;
#6934=VECTOR ( 'NONE', #3643, 1000.000000000000114 ) ;
#6935=AXIS2_PLACEMENT_3D ( 'NONE', #7300, #12240, #12297 ) ;
#6937=DIRECTION ( 'NONE',  ( 0.000000000000000000, 1.000000000000000000, 0.000000000000000000 ) ) ;
#6945=ORIENTED_EDGE ( 'NONE', *, *, #12004, .F. ) ;
#6948=CARTESIAN_POINT ( 'NONE',  ( 153.9282213272189495, -30.00000000000000000, 245.7765299597151341 ) ) ;
#6953=VERTEX_POINT ( 'NONE', #2701 ) ;
#6957=VERTEX_POINT ( 'NONE', #6597 ) ;
#6961=ORIENTED_EDGE ( 'NONE', *, *, #8372, .F. ) ;
#6966=FACE_OUTER_BOUND ( 'NONE', #12715, .T. ) ;
#6973=EDGE_CURVE ( 'NONE', #237, #12419, #12453, .T. ) ;
#6986=EDGE_LOOP ( 'NONE', ( #8437, #9052, #5878, #3450 ) ) ;
#6987=VERTEX_POINT ( 'NONE', #4513 ) ;
#6989=EDGE_LOOP ( 'NONE', ( #3284, #11899, #4607, #8645 ) ) ;
#6993=DIRECTION ( 'NONE',  ( -0.000000000000000000, -1.000000000000000000, 0.000000000000000000 ) ) ;
#7003=VECTOR ( 'NONE', #2023, 1000.000000000000000 ) ;
#7004=DIRECTION ( 'NONE',  ( 0.6368676505102716101, 0.000000000000000000, 0.7709731485165527420 ) ) ;
#7014=CARTESIAN_POINT ( 'NONE',  ( -27.68945685411286561, -30.00000000000000000, 290.6841825403027997 ) ) ;
#7024=EDGE_CURVE ( 'NONE', #1244, #1953, #10100, .T. ) ;
#7025=AXIS2_PLACEMENT_3D ( 'NONE', #9574, #1447, #10710 ) ;
#7026=CARTESIAN_POINT ( 'NONE',  ( 157.1762463448213225, -19.40000000000000213, 249.7084930171495500 ) ) ;
#7034=EDGE_CURVE ( 'NONE', #12935, #11832, #10651, .T. ) ;
#7035=VERTEX_POINT ( 'NONE', #8786 ) ;
#7037=ORIENTED_EDGE ( 'NONE', *, *, #7552, .F. ) ;
#7038=VECTOR ( 'NONE', #6614, 1000.000000000000000 ) ;
#7052=LINE ( 'NONE', #12181, #8802 ) ;
#7053=CIRCLE ( 'NONE', #7362, 6.500000000000005329 ) ;
#7054=ORIENTED_EDGE ( 'NONE', *, *, #12232, .F. ) ;
#7058=EDGE_LOOP ( 'NONE', ( #5674, #2473 ) ) ;
#7061=DIRECTION ( 'NONE',  ( 0.6368676505102737195, 0.000000000000000000, 0.7709731485165509657 ) ) ;
#7064=CIRCLE ( 'NONE', #11625, 5.499999999999986677 ) ;
#7067=DIRECTION ( 'NONE',  ( -0.000000000000000000, -1.000000000000000000, 0.000000000000000000 ) ) ;
#7081=AXIS2_PLACEMENT_3D ( 'NONE', #2282, #4216, #11560 ) ;
#7084=ORIENTED_EDGE ( 'NONE', *, *, #7989, .T. ) ;
#7085=AXIS2_PLACEMENT_3D ( 'NONE', #509, #12695, #7629 ) ;
#7088=EDGE_LOOP ( 'NONE', ( #12480, #4144, #6304, #1761 ) ) ;
#7089=ORIENTED_EDGE ( 'NONE', *, *, #5583, .F. ) ;
#7090=DIRECTION ( 'NONE',  ( -0.000000000000000000, -1.000000000000000000, 0.000000000000000000 ) ) ;
#7091=FACE_OUTER_BOUND ( 'NONE', #4896, .T. ) ;
#7094=AXIS2_PLACEMENT_3D ( 'NONE', #11311, #12573, #10699 ) ;
#7100=EDGE_CURVE ( 'NONE', #11817, #2751, #7052, .T. ) ;
#7104=CIRCLE ( 'NONE', #3044, 6.500000000000005329 ) ;
#7110=CARTESIAN_POINT ( 'NONE',  ( -289.8128292627096130, -28.60000000000000142, 10.41748504886635907 ) ) ;
#7112=CARTESIAN_POINT ( 'NONE',  ( 0.000000000000000000, 0.000000000000000000, 0.000000000000000000 ) ) ;
#7113=CARTESIAN_POINT ( 'NONE',  ( -24.18668477630637526, -30.00000000000000000, 294.9245348571438967 ) ) ;
#7115=DIRECTION ( 'NONE',  ( 0.4503334343941555740, 0.7071067811865490160, 0.5451603414287971017 ) ) ;
#7125=TOROIDAL_SURFACE ( 'NONE', #3066, 261.5294117647060261, 2.000000000000000000 ) ;
#7141=ORIENTED_EDGE ( 'NONE', *, *, #12585, .F. ) ;
#7144=ADVANCED_FACE ( 'NONE', ( #9112 ), #9050, .F. ) ;
#7149=DIRECTION ( 'NONE',  ( 0.6368676505102706109, 0.000000000000000000, 0.7709731485165535192 ) ) ;
#7154=ORIENTED_EDGE ( 'NONE', *, *, #11353, .T. ) ;
#7162=DIRECTION ( 'NONE',  ( -0.4503334343941575724, 0.7071067811865460184, -0.5451603414287993221 ) ) ;
#7165=VERTEX_POINT ( 'NONE', #4305 ) ;
#7167=ORIENTED_EDGE ( 'NONE', *, *, #7614, .T. ) ;
#7171=DIRECTION ( 'NONE',  ( -0.000000000000000000, -1.000000000000000000, 0.000000000000000000 ) ) ;
#7175=CONICAL_SURFACE ( 'NONE', #1429, 5.499999999999986677, 0.7853981633974461696 ) ;
#7176=DIRECTION ( 'NONE',  ( -0.000000000000000000, -1.000000000000000000, 0.000000000000000000 ) ) ;
#7184=CARTESIAN_POINT ( 'NONE',  ( 27.68945685411497593, -18.00000000000000000, -290.6841825403026291 ) ) ;
#7189=DIRECTION ( 'NONE',  ( 0.6368676505102707219, 0.000000000000000000, 0.7709731485165535192 ) ) ;
#7191=AXIS2_PLACEMENT_3D ( 'NONE', #2780, #4651, #1734 ) ;
#7207=VECTOR ( 'NONE', #2277, 1000.000000000000000 ) ;
#7211=DIRECTION ( 'NONE',  ( 0.6368676505102698338, 0.000000000000000000, 0.7709731485165542964 ) ) ;
#7214=ADVANCED_FACE ( 'NONE', ( #2107 ), #6681, .F. ) ;
#7218=ADVANCED_FACE ( 'NONE', ( #12507 ), #5605, .F. ) ;
#7219=ORIENTED_EDGE ( 'NONE', *, *, #12422, .F. ) ;
#7221=DIRECTION ( 'NONE',  ( -0.000000000000000000, -1.000000000000000000, 0.000000000000000000 ) ) ;
#7231=DIRECTION ( 'NONE',  ( 0.6368676505102709440, 0.000000000000000000, 0.7709731485165532971 ) ) ;
#7238=EDGE_LOOP ( 'NONE', ( #3617, #5904, #2017, #2771 ) ) ;
#7239=CARTESIAN_POINT ( 'NONE',  ( 139.1326329530957082, -30.00000000000000000, -252.2620519511468729 ) ) ;
#7241=ORIENTED_EDGE ( 'NONE', *, *, #12673, .F. ) ;
#7242=DIRECTION ( 'NONE',  ( 0.000000000000000000, 1.000000000000000000, 0.000000000000000000 ) ) ;
#7244=DIRECTION ( 'NONE',  ( 0.6368676505102707219, 0.000000000000000000, 0.7709731485165536302 ) ) ;
#7245=DIRECTION ( 'NONE',  ( -0.000000000000000000, -1.000000000000000000, 0.000000000000000000 ) ) ;
#7246=LINE ( 'NONE', #9175, #6491 ) ;
#7247=CARTESIAN_POINT ( 'NONE',  ( -290.6841825403030839, -19.00000000000000000, -27.68945685411394919 ) ) ;
#7256=ORIENTED_EDGE ( 'NONE', *, *, #12017, .F. ) ;
#7266=CARTESIAN_POINT ( 'NONE',  ( -160.6180214586902650, 11.79660968244693997, -194.4394280558747710 ) ) ;
#7267=ADVANCED_FACE ( 'NONE', ( #7317 ), #11384, .F. ) ;
#7273=LINE ( 'NONE', #11467, #6483 ) ;
#7280=CARTESIAN_POINT ( 'NONE',  ( 290.6841825403032544, -19.00000000000000000, 27.68945685411186730 ) ) ;
#7283=AXIS2_PLACEMENT_3D ( 'NONE', #2591, #1536, #6610 ) ;
#7288=DIRECTION ( 'NONE',  ( -0.000000000000000000, -1.000000000000000000, 0.000000000000000000 ) ) ;
#7300=CARTESIAN_POINT ( 'NONE',  ( -289.8128292627096130, -18.00000000000000000, 10.41748504886635907 ) ) ;
#7301=ORIENTED_EDGE ( 'NONE', *, *, #1156, .T. ) ;
#7305=DIRECTION ( 'NONE',  ( 0.6368676505102689456, 0.000000000000000000, 0.7709731485165549625 ) ) ;
#7312=AXIS2_PLACEMENT_3D ( 'NONE', #7889, #8691, #11705 ) ;
#7317=FACE_OUTER_BOUND ( 'NONE', #663, .T. ) ;
#7318=ORIENTED_EDGE ( 'NONE', *, *, #8372, .T. ) ;
#7328=LINE ( 'NONE', #4126, #3082 ) ;
#7331=AXIS2_PLACEMENT_3D ( 'NONE', #5033, #11109, #3099 ) ;
#7333=DIRECTION ( 'NONE',  ( 0.6368676505102709440, 0.000000000000000000, 0.7709731485165532971 ) ) ;
#7341=LINE ( 'NONE', #8219, #2 ) ;
#7343=FACE_OUTER_BOUND ( 'NONE', #5169, .T. ) ;
#7344=FACE_OUTER_BOUND ( 'NONE', #9150, .T. ) ;
#7354=VERTEX_POINT ( 'NONE', #8769 ) ;
#7355=CARTESIAN_POINT ( 'NONE',  ( 159.6627199829248411, -25.00000000000000000, 193.2829683331000012 ) ) ;
#7362=AXIS2_PLACEMENT_3D ( 'NONE', #233, #4292, #8374 ) ;
#7367=ORIENTED_EDGE ( 'NONE', *, *, #11245, .T. ) ;
#7368=ADVANCED_FACE ( 'NONE', ( #5701 ), #4622, .F. ) ;
#7374=DIRECTION ( 'NONE',  ( -0.000000000000000000, -1.000000000000000000, 0.000000000000000000 ) ) ;
#7383=DIRECTION ( 'NONE',  ( -0.6368676505102707219, 0.000000000000000000, -0.7709731485165535192 ) ) ;
#7385=EDGE_LOOP ( 'NONE', ( #27, #8837 ) ) ;
#7394=DIRECTION ( 'NONE',  ( -0.6368676505102700558, 0.000000000000000000, -0.7709731485165541853 ) ) ;
#7404=DIRECTION ( 'NONE',  ( -0.000000000000000000, -1.000000000000000000, 0.000000000000000000 ) ) ;
#7406=VERTEX_POINT ( 'NONE', #9507 ) ;
#7409=EDGE_CURVE ( 'NONE', #5526, #3236, #294, .T. ) ;
#7410=DIRECTION ( 'NONE',  ( 0.6368676505102737195, 0.000000000000000000, 0.7709731485165509657 ) ) ;
#7426=CIRCLE ( 'NONE', #1679, 5.500000000000015099 ) ;
#7430=ORIENTED_EDGE ( 'NONE', *, *, #2712, .T. ) ;
#7431=ORIENTED_EDGE ( 'NONE', *, *, #11711, .F. ) ;
#7434=FACE_OUTER_BOUND ( 'NONE', #10725, .T. ) ;
#7436=EDGE_CURVE ( 'NONE', #3272, #11832, #7104, .T. ) ;
#7444=DIRECTION ( 'NONE',  ( 0.6368676505102707219, 0.000000000000000000, 0.7709731485165535192 ) ) ;
#7450=ORIENTED_EDGE ( 'NONE', *, *, #11353, .F. ) ;
#7463=ADVANCED_FACE ( 'NONE', ( #6518 ), #4747, .F. ) ;
#7469=DIRECTION ( 'NONE',  ( 0.000000000000000000, 1.000000000000000000, 0.000000000000000000 ) ) ;
#7471=EDGE_LOOP ( 'NONE', ( #12950, #1079, #7785, #1795 ) ) ;
#7476=DIRECTION ( 'NONE',  ( -0.000000000000000000, -1.000000000000000000, 0.000000000000000000 ) ) ;
#7478=LINE ( 'NONE', #3134, #1077 ) ;
#7481=CIRCLE ( 'NONE', #7025, 5.500000000000007994 ) ;
#7483=ORIENTED_EDGE ( 'NONE', *, *, #12569, .T. ) ;
#7485=CYLINDRICAL_SURFACE ( 'NONE', #604, 5.500000000000015099 ) ;
#7486=FACE_BOUND ( 'NONE', #5104, .T. ) ;
#7489=ORIENTED_EDGE ( 'NONE', *, *, #12302, .F. ) ;
#7497=ORIENTED_EDGE ( 'NONE', *, *, #5468, .F. ) ;
#7500=EDGE_LOOP ( 'NONE', ( #8616, #12609, #1193, #7489 ) ) ;
#7501=VECTOR ( 'NONE', #1736, 1000.000000000000000 ) ;
#7503=CARTESIAN_POINT ( 'NONE',  ( 290.6841825403032544, -18.00000000000000000, 27.68945685411186730 ) ) ;
#7507=DIRECTION ( 'NONE',  ( 0.6368676505102716101, 0.000000000000000000, 0.7709731485165527420 ) ) ;
#7512=AXIS2_PLACEMENT_3D ( 'NONE', #5425, #6428, #3339 ) ;
#7514=CIRCLE ( 'NONE', #11562, 5.499999999999986677 ) ;
#7518=DIRECTION ( 'NONE',  ( -0.4503334343941627904, -0.7071067811865381358, -0.5451603414288054283 ) ) ;
#7528=ADVANCED_FACE ( 'NONE', ( #4761 ), #5830, .F. ) ;
#7531=ORIENTED_EDGE ( 'NONE', *, *, #2315, .T. ) ;
#7533=DIRECTION ( 'NONE',  ( -0.000000000000000000, -1.000000000000000000, 0.000000000000000000 ) ) ;
#7534=CARTESIAN_POINT ( 'NONE',  ( 221.6213872890270977, -29.00000000000000000, -190.2057062658400923 ) ) ;
#7538=CONICAL_SURFACE ( 'NONE', #3485, 6.500000000000005329, 0.7853981633974518317 ) ;
#7539=DIRECTION ( 'NONE',  ( -0.000000000000000000, -1.000000000000000000, 0.000000000000000000 ) ) ;
#7543=AXIS2_PLACEMENT_3D ( 'NONE', #7833, #8651, #2634 ) ;
#7547=ORIENTED_EDGE ( 'NONE', *, *, #8205, .F. ) ;
#7548=EDGE_LOOP ( 'NONE', ( #8199, #2179, #4534, #10020 ) ) ;
#7552=EDGE_CURVE ( 'NONE', #10483, #9653, #9964, .T. ) ;
#7558=TOROIDAL_SURFACE ( 'NONE', #8619, 252.1999999999999886, 2.000000000000000000 ) ;
#7567=VECTOR ( 'NONE', #5227, 1000.000000000000000 ) ;
#7569=CYLINDRICAL_SURFACE ( 'NONE', #6061, 305.0000000000000000 ) ;
#7585=DIRECTION ( 'NONE',  ( 0.6368676505102707219, 0.000000000000000000, 0.7709731485165535192 ) ) ;
#7594=CARTESIAN_POINT ( 'NONE',  ( 185.9653539490014111, -19.00000000000000000, 225.1241593668316625 ) ) ;
#7597=EDGE_CURVE ( 'NONE', #2539, #11365, #9036, .T. ) ;
#7605=VECTOR ( 'NONE', #1661, 999.9999999999998863 ) ;
#7607=ORIENTED_EDGE ( 'NONE', *, *, #10355, .F. ) ;
#7610=CARTESIAN_POINT ( 'NONE',  ( 190.1049936773181628, -30.00000000000000000, 230.1354848321892632 ) ) ;
#7613=( GEOMETRIC_REPRESENTATION_CONTEXT ( 3 ) GLOBAL_UNCERTAINTY_ASSIGNED_CONTEXT ( ( #2899 ) ) GLOBAL_UNIT_ASSIGNED_CONTEXT ( ( #10895, #3893, #1771 ) ) REPRESENTATION_CONTEXT ( 'NONE', 'WORKASPACE' ) );
#7614=EDGE_CURVE ( 'NONE', #10097, #2361, #12901, .T. ) ;
#7621=ADVANCED_FACE ( 'NONE', ( #4026 ), #7538, .F. ) ;
#7624=ORIENTED_EDGE ( 'NONE', *, *, #5432, .T. ) ;
#7627=DIRECTION ( 'NONE',  ( 0.6368676505102707219, 0.000000000000000000, 0.7709731485165535192 ) ) ;
#7629=DIRECTION ( 'NONE',  ( 0.6368676505102716101, 0.000000000000000000, 0.7709731485165527420 ) ) ;
#7630=ADVANCED_FACE ( 'NONE', ( #2748 ), #96, .F. ) ;
#7633=AXIS2_PLACEMENT_3D ( 'NONE', #11255, #6195, #1196 ) ;
#7642=CARTESIAN_POINT ( 'NONE',  ( -294.1869546181095529, -30.00000000000000000, -31.92980917095498938 ) ) ;
#7647=DIRECTION ( 'NONE',  ( 0.6368676505102707219, 0.000000000000000000, 0.7709731485165535192 ) ) ;
#7662=ADVANCED_FACE ( 'NONE', ( #837 ), #2830, .F. ) ;
#7663=DIRECTION ( 'NONE',  ( -0.000000000000000000, -1.000000000000000000, 0.000000000000000000 ) ) ;
#7670=ORIENTED_EDGE ( 'NONE', *, *, #10595, .F. ) ;
#7674=DIRECTION ( 'NONE',  ( -0.6368676505102708330, 0.000000000000000000, -0.7709731485165536302 ) ) ;
#7677=DIRECTION ( 'NONE',  ( -0.6368676505102689456, 0.000000000000000000, -0.7709731485165549625 ) ) ;
#7682=EDGE_LOOP ( 'NONE', ( #6926, #4375 ) ) ;
#7684=DIRECTION ( 'NONE',  ( -0.6368676505102690566, 0.000000000000000000, -0.7709731485165549625 ) ) ;
#7685=ORIENTED_EDGE ( 'NONE', *, *, #1723, .F. ) ;
#7689=EDGE_CURVE ( 'NONE', #9991, #2838, #9298, .T. ) ;
#7695=DIRECTION ( 'NONE',  ( 0.000000000000000000, 1.000000000000000000, 0.000000000000000000 ) ) ;
#7699=CARTESIAN_POINT ( 'NONE',  ( 135.8846079354933352, -30.00000000000000000, -256.1940150085812888 ) ) ;
#7700=EDGE_LOOP ( 'NONE', ( #11827, #10871, #8857, #401 ) ) ;
#7702=VERTEX_POINT ( 'NONE', #12367 ) ;
#7705=DIRECTION ( 'NONE',  ( -0.000000000000000000, -1.000000000000000000, 0.000000000000000000 ) ) ;
#7706=FACE_BOUND ( 'NONE', #1581, .T. ) ;
#7709=CARTESIAN_POINT ( 'NONE',  ( 185.9653539490014111, -29.00000000000000000, 225.1241593668316625 ) ) ;
#7718=ORIENTED_EDGE ( 'NONE', *, *, #6859, .F. ) ;
#7720=ORIENTED_EDGE ( 'NONE', *, *, #864, .F. ) ;
#7728=FACE_OUTER_BOUND ( 'NONE', #4679, .T. ) ;
#7734=CONICAL_SURFACE ( 'NONE', #10926, 5.500000000000015099, 0.7853981633974461696 ) ;
#7753=AXIS2_PLACEMENT_3D ( 'NONE', #8575, #6380, #10438 ) ;
#7756=ORIENTED_EDGE ( 'NONE', *, *, #10963, .F. ) ;
#7760=CARTESIAN_POINT ( 'NONE',  ( 24.18668477630848557, -19.00000000000000000, -294.9245348571437262 ) ) ;
#7766=EDGE_CURVE ( 'NONE', #8820, #1725, #9027, .T. ) ;
#7770=ORIENTED_EDGE ( 'NONE', *, *, #11589, .T. ) ;
#7773=CARTESIAN_POINT ( 'NONE',  ( 23.54981712579822073, -18.00000000000000000, -295.6955080056602583 ) ) ;
#7774=DIRECTION ( 'NONE',  ( -0.000000000000000000, -1.000000000000000000, 0.000000000000000000 ) ) ;
#7785=ORIENTED_EDGE ( 'NONE', *, *, #8459, .T. ) ;
#7787=DIRECTION ( 'NONE',  ( -0.000000000000000000, -1.000000000000000000, 0.000000000000000000 ) ) ;
#7808=CARTESIAN_POINT ( 'NONE',  ( -24.18668477630637526, -19.00000000000000000, 294.9245348571438967 ) ) ;
#7813=ORIENTED_EDGE ( 'NONE', *, *, #4064, .T. ) ;
#7818=CIRCLE ( 'NONE', #5481, 6.500000000000005329 ) ;
#7820=CARTESIAN_POINT ( 'NONE',  ( 139.1326329530957082, -19.40000000000000213, -252.2620519511468729 ) ) ;
#7826=DIRECTION ( 'NONE',  ( 0.6368676505102716101, 0.000000000000000000, 0.7709731485165527420 ) ) ;
#7828=ORIENTED_EDGE ( 'NONE', *, *, #446, .F. ) ;
#7831=EDGE_CURVE ( 'NONE', #1100, #6702, #3263, .T. ) ;
#7833=CARTESIAN_POINT ( 'NONE',  ( 27.68945685411497593, -30.00000000000000000, -290.6841825403026291 ) ) ;
#7838=VECTOR ( 'NONE', #3062, 1000.000000000000000 ) ;
#7844=VERTEX_POINT ( 'NONE', #8476 ) ;
#7847=EDGE_LOOP ( 'NONE', ( #5742, #3072, #8320, #10754 ) ) ;
#7854=CIRCLE ( 'NONE', #2103, 250.1999999999999602 ) ;
#7869=ORIENTED_EDGE ( 'NONE', *, *, #2754, .T. ) ;
#7874=VECTOR ( 'NONE', #2306, 1000.000000000000000 ) ;
#7880=EDGE_LOOP ( 'NONE', ( #4362, #11015, #8500, #6961 ) ) ;
#7889=CARTESIAN_POINT ( 'NONE',  ( -185.9653539489998195, -30.00000000000000000, -225.1241593668329699 ) ) ;
#7891=CARTESIAN_POINT ( 'NONE',  ( 0.000000000000000000, 2.772967769358929857, 0.000000000000000000 ) ) ;
#7892=DIRECTION ( 'NONE',  ( 0.4503334343941555740, 0.7071067811865490160, 0.5451603414287971017 ) ) ;
#7893=LINE ( 'NONE', #4756, #5597 ) ;
#7895=DIRECTION ( 'NONE',  ( 0.000000000000000000, 1.000000000000000000, 0.000000000000000000 ) ) ;
#7903=LINE ( 'NONE', #12041, #10212 ) ;
#7905=CARTESIAN_POINT ( 'NONE',  ( 290.6841825403032544, -18.00000000000000000, 27.68945685411186730 ) ) ;
#7917=ORIENTED_EDGE ( 'NONE', *, *, #986, .T. ) ;
#7918=ORIENTED_EDGE ( 'NONE', *, *, #9725, .F. ) ;
#7923=FACE_OUTER_BOUND ( 'NONE', #4662, .T. ) ;
#7926=LINE ( 'NONE', #6933, #8671 ) ;
#7934=ADVANCED_FACE ( 'NONE', ( #7343 ), #3054, .F. ) ;
#7936=CIRCLE ( 'NONE', #11778, 6.500000000000026645 ) ;
#7940=ORIENTED_EDGE ( 'NONE', *, *, #5957, .F. ) ;
#7944=VECTOR ( 'NONE', #3620, 1000.000000000000114 ) ;
#7953=ORIENTED_EDGE ( 'NONE', *, *, #5173, .T. ) ;
#7958=ORIENTED_EDGE ( 'NONE', *, *, #12873, .F. ) ;
#7969=ORIENTED_EDGE ( 'NONE', *, *, #6119, .F. ) ;
#7970=DIRECTION ( 'NONE',  ( 0.000000000000000000, 1.000000000000000000, 0.000000000000000000 ) ) ;
#7971=ORIENTED_EDGE ( 'NONE', *, *, #6555, .F. ) ;
#7975=VECTOR ( 'NONE', #4755, 1000.000000000000000 ) ;
#7977=CARTESIAN_POINT ( 'NONE',  ( -159.3442861576697283, 0.000000000000000000, -192.8974817588416499 ) ) ;
#7979=DIRECTION ( 'NONE',  ( -0.000000000000000000, -1.000000000000000000, 0.000000000000000000 ) ) ;
#7989=EDGE_CURVE ( 'NONE', #366, #2919, #11340, .T. ) ;
#7992=ORIENTED_EDGE ( 'NONE', *, *, #4667, .F. ) ;
#7997=DIRECTION ( 'NONE',  ( -0.000000000000000000, -1.000000000000000000, 0.000000000000000000 ) ) ;
#8003=DIRECTION ( 'NONE',  ( -0.000000000000000000, -1.000000000000000000, 0.000000000000000000 ) ) ;
#8017=DIRECTION ( 'NONE',  ( -0.000000000000000000, -1.000000000000000000, 0.000000000000000000 ) ) ;
#8024=CYLINDRICAL_SURFACE ( 'NONE', #11478, 254.1999999999999886 ) ;
#8025=CARTESIAN_POINT ( 'NONE',  ( 166.5596220099214406, -3.327561323230905366, 201.6321540179175997 ) ) ;
#8026=ADVANCED_FACE ( 'NONE', ( #10472 ), #4346, .F. ) ;
#8032=ADVANCED_FACE ( 'NONE', ( #3390 ), #12014, .T. ) ;
#8033=ORIENTED_EDGE ( 'NONE', *, *, #11828, .F. ) ;
#8040=FACE_OUTER_BOUND ( 'NONE', #4707, .T. ) ;
#8058=DIRECTION ( 'NONE',  ( 0.6368676505102708330, 0.000000000000000000, 0.7709731485165535192 ) ) ;
#8059=DIRECTION ( 'NONE',  ( -0.000000000000000000, -1.000000000000000000, 0.000000000000000000 ) ) ;
#8071=AXIS2_PLACEMENT_3D ( 'NONE', #11670, #9784, #1659 ) ;
#8072=VERTEX_POINT ( 'NONE', #6608 ) ;
#8073=VECTOR ( 'NONE', #2392, 1000.000000000000114 ) ;
#8080=CARTESIAN_POINT ( 'NONE',  ( -159.6627199829248696, -25.00000000000000000, -193.2829683330999728 ) ) ;
#8081=LINE ( 'NONE', #2997, #10271 ) ;
#8082=AXIS2_PLACEMENT_3D ( 'NONE', #10083, #6153, #2871 ) ;
#8089=CIRCLE ( 'NONE', #2960, 270.0000000000000000 ) ;
#8095=DIRECTION ( 'NONE',  ( -0.000000000000000000, -1.000000000000000000, 0.000000000000000000 ) ) ;
#8104=EDGE_CURVE ( 'NONE', #9851, #237, #7246, .T. ) ;
#8106=EDGE_CURVE ( 'NONE', #8628, #4466, #4766, .T. ) ;
#8109=ORIENTED_EDGE ( 'NONE', *, *, #6060, .T. ) ;
#8116=DIRECTION ( 'NONE',  ( 0.6368676505102689456, 0.000000000000000000, 0.7709731485165549625 ) ) ;
#8123=EDGE_CURVE ( 'NONE', #8455, #11555, #10106, .T. ) ;
#8129=EDGE_CURVE ( 'NONE', #5922, #8469, #9885, .T. ) ;
#8130=AXIS2_PLACEMENT_3D ( 'NONE', #8975, #11786, #10839 ) ;
#8132=DIRECTION ( 'NONE',  ( 0.000000000000000000, 1.000000000000000000, 0.000000000000000000 ) ) ;
#8141=DIRECTION ( 'NONE',  ( -0.000000000000000000, -1.000000000000000000, 0.000000000000000000 ) ) ;
#8142=EDGE_LOOP ( 'NONE', ( #9873, #3720, #11637, #7547 ) ) ;
#8143=ORIENTED_EDGE ( 'NONE', *, *, #8106, .F. ) ;
#8150=CYLINDRICAL_SURFACE ( 'NONE', #3673, 5.500000000000015099 ) ;
#8161=ORIENTED_EDGE ( 'NONE', *, *, #10480, .F. ) ;
#8162=CARTESIAN_POINT ( 'NONE',  ( -185.9653539489998195, -30.00000000000000000, -225.1241593668329699 ) ) ;
#8183=EDGE_CURVE ( 'NONE', #10082, #12948, #1913, .T. ) ;
#8187=DIRECTION ( 'NONE',  ( 0.4503334343941581830, -0.7071067811865450192, 0.5451603414288000993 ) ) ;
#8199=ORIENTED_EDGE ( 'NONE', *, *, #5432, .F. ) ;
#8202=CARTESIAN_POINT ( 'NONE',  ( -0.000000000000000000, -19.00000000000000000, 0.000000000000000000 ) ) ;
#8205=EDGE_CURVE ( 'NONE', #6789, #2094, #12443, .T. ) ;
#8206=AXIS2_PLACEMENT_3D ( 'NONE', #7280, #7476, #2341 ) ;
#8207=DIRECTION ( 'NONE',  ( -0.000000000000000000, -1.000000000000000000, 0.000000000000000000 ) ) ;
#8215=VECTOR ( 'NONE', #6013, 1000.000000000000000 ) ;
#8217=CYLINDRICAL_SURFACE ( 'NONE', #4862, 5.100000000000003197 ) ;
#8219=CARTESIAN_POINT ( 'NONE',  ( 31.82909658243173467, -30.00000000000000000, -285.6728570749450569 ) ) ;
#8221=CARTESIAN_POINT ( 'NONE',  ( 228.6269314446401211, -29.00000000000000000, -181.7250016321579835 ) ) ;
#8222=CARTESIAN_POINT ( 'NONE',  ( 0.000000000000000000, 20.00000000000000000, 0.000000000000000000 ) ) ;
#8225=AXIS2_PLACEMENT_3D ( 'NONE', #12847, #10523, #4445 ) ;
#8227=VERTEX_POINT ( 'NONE', #10569 ) ;
#8242=LINE ( 'NONE', #7239, #1189 ) ;
#8248=ADVANCED_FACE ( 'NONE', ( #11642 ), #7569, .T. ) ;
#8249=ADVANCED_FACE ( 'NONE', ( #2372 ), #1437, .T. ) ;
#8250=FACE_OUTER_BOUND ( 'NONE', #7088, .T. ) ;
#8252=DIRECTION ( 'NONE',  ( -0.000000000000000000, -1.000000000000000000, 0.000000000000000000 ) ) ;
#8257=EDGE_LOOP ( 'NONE', ( #3366, #514, #1250, #8986 ) ) ;
#8258=CARTESIAN_POINT ( 'NONE',  ( 0.000000000000000000, 0.000000000000000000, 0.000000000000000000 ) ) ;
#8262=ORIENTED_EDGE ( 'NONE', *, *, #10275, .F. ) ;
#8279=CARTESIAN_POINT ( 'NONE',  ( -290.6841825403030839, -18.00000000000000000, -27.68945685411394919 ) ) ;
#8281=CONICAL_SURFACE ( 'NONE', #1456, 5.500000000000015099, 0.7853981633974461696 ) ;
#8298=VERTEX_POINT ( 'NONE', #2240 ) ;
#8310=ORIENTED_EDGE ( 'NONE', *, *, #2134, .F. ) ;
#8316=DIRECTION ( 'NONE',  ( -0.4503334343941556295, 0.7071067811865489050, -0.5451603414287969906 ) ) ;
#8320=ORIENTED_EDGE ( 'NONE', *, *, #1973, .T. ) ;
#8325=EDGE_CURVE ( 'NONE', #4274, #823, #4299, .T. ) ;
#8329=ORIENTED_EDGE ( 'NONE', *, *, #12032, .F. ) ;
#8332=CYLINDRICAL_SURFACE ( 'NONE', #7633, 5.500000000000015099 ) ;
#8334=EDGE_CURVE ( 'NONE', #7035, #3038, #12933, .T. ) ;
#8340=ORIENTED_EDGE ( 'NONE', *, *, #5260, .F. ) ;
#8342=ORIENTED_EDGE ( 'NONE', *, *, #2924, .F. ) ;
#8344=CARTESIAN_POINT ( 'NONE',  ( 225.1241593668336236, -19.00000000000000000, -185.9653539489990521 ) ) ;
#8348=ADVANCED_FACE ( 'NONE', ( #11895 ), #2009, .F. ) ;
#8367=CIRCLE ( 'NONE', #10903, 250.1999999999999602 ) ;
#8372=EDGE_CURVE ( 'NONE', #2275, #6648, #12862, .T. ) ;
#8374=DIRECTION ( 'NONE',  ( 0.6368676505102716101, 0.000000000000000000, 0.7709731485165527420 ) ) ;
#8376=ORIENTED_EDGE ( 'NONE', *, *, #12569, .F. ) ;
#8381=DIRECTION ( 'NONE',  ( 0.6368676505102716101, 0.000000000000000000, 0.7709731485165527420 ) ) ;
#8387=AXIS2_PLACEMENT_3D ( 'NONE', #10533, #12467, #11672 ) ;
#8391=CARTESIAN_POINT ( 'NONE',  ( -194.2446334056326123, -19.00000000000000000, -235.1468102975487682 ) ) ;
#8393=ORIENTED_EDGE ( 'NONE', *, *, #140, .F. ) ;
#8394=VECTOR ( 'NONE', #6170, 1000.000000000000000 ) ;
#8400=DIRECTION ( 'NONE',  ( 0.6368676505102707219, 0.000000000000000000, 0.7709731485165535192 ) ) ;
#8408=FACE_OUTER_BOUND ( 'NONE', #4402, .T. ) ;
#8415=DIRECTION ( 'NONE',  ( 0.6368676505102695007, 0.000000000000000000, 0.7709731485165545184 ) ) ;
#8425=EDGE_CURVE ( 'NONE', #3933, #4419, #2815, .T. ) ;
#8426=DIRECTION ( 'NONE',  ( -0.000000000000000000, -1.000000000000000000, 0.000000000000000000 ) ) ;
#8427=PLANE ( 'NONE',  #9972 ) ;
#8430=AXIS2_PLACEMENT_3D ( 'NONE', #8783, #6661, #10719 ) ;
#8431=DIRECTION ( 'NONE',  ( 0.6368676505102695007, 0.000000000000000000, 0.7709731485165545184 ) ) ;
#8433=CIRCLE ( 'NONE', #2660, 254.1999999999999886 ) ;
#8437=ORIENTED_EDGE ( 'NONE', *, *, #9245, .F. ) ;
#8438=DIRECTION ( 'NONE',  ( -0.000000000000000000, -1.000000000000000000, 0.000000000000000000 ) ) ;
#8453=ORIENTED_EDGE ( 'NONE', *, *, #5225, .T. ) ;
#8455=VERTEX_POINT ( 'NONE', #7820 ) ;
#8459=EDGE_CURVE ( 'NONE', #2079, #11730, #706, .T. ) ;
#8469=VERTEX_POINT ( 'NONE', #4689 ) ;
#8473=DIRECTION ( 'NONE',  ( -0.7709731485165534082, 0.000000000000000000, 0.6368676505102708330 ) ) ;
#8476=CARTESIAN_POINT ( 'NONE',  ( 294.8238222686200061, -30.00000000000000000, 32.70078231946946090 ) ) ;
#8483=ORIENTED_EDGE ( 'NONE', *, *, #11661, .F. ) ;
#8484=ADVANCED_FACE ( 'NONE', ( #12696 ), #3926, .F. ) ;
#8487=CARTESIAN_POINT ( 'NONE',  ( 0.000000000000000000, 11.79660968244693997, 0.000000000000000000 ) ) ;
#8488=FACE_BOUND ( 'NONE', #5036, .T. ) ;
#8490=AXIS2_PLACEMENT_3D ( 'NONE', #8344, #12466, #206 ) ;
#8495=CARTESIAN_POINT ( 'NONE',  ( 132.6365829178909621, -19.40000000000000213, -260.1259780660157048 ) ) ;
#8500=ORIENTED_EDGE ( 'NONE', *, *, #5328, .T. ) ;
#8501=DIRECTION ( 'NONE',  ( 0.4503334343941595153, -0.7071067811865431318, 0.5451603414288016536 ) ) ;
#8502=EDGE_LOOP ( 'NONE', ( #12816, #10816, #5152, #11954 ) ) ;
#8504=CIRCLE ( 'NONE', #10189, 259.6078431372549744 ) ;
#8506=CARTESIAN_POINT ( 'NONE',  ( 135.8846079354933352, -30.00000000000000000, -256.1940150085812888 ) ) ;
#8507=LINE ( 'NONE', #239, #6815 ) ;
#8508=CARTESIAN_POINT ( 'NONE',  ( -286.5648042451072115, -28.60000000000000142, 14.34944810630077505 ) ) ;
#8510=CARTESIAN_POINT ( 'NONE',  ( 294.1869546181097235, -29.00000000000000000, 31.92980917095288618 ) ) ;
#8513=AXIS2_PLACEMENT_3D ( 'NONE', #3203, #1216, #11349 ) ;
#8515=VERTEX_POINT ( 'NONE', #100 ) ;
#8516=DIRECTION ( 'NONE',  ( -0.000000000000000000, -1.000000000000000000, 0.000000000000000000 ) ) ;
#8519=FACE_OUTER_BOUND ( 'NONE', #1613, .T. ) ;
#8520=AXIS2_PLACEMENT_3D ( 'NONE', #12341, #9138, #15 ) ;
#8525=CARTESIAN_POINT ( 'NONE',  ( -193.6077657551222728, -30.00000000000000000, -234.3758371490322645 ) ) ;
#8526=DIRECTION ( 'NONE',  ( 0.6368676505102707219, 0.000000000000000000, 0.7709731485165535192 ) ) ;
#8527=ADVANCED_FACE ( 'NONE', ( #9032 ), #6231, .F. ) ;
#8533=EDGE_CURVE ( 'NONE', #9382, #10885, #5148, .T. ) ;
#8536=ORIENTED_EDGE ( 'NONE', *, *, #12084, .T. ) ;
#8538=CARTESIAN_POINT ( 'NONE',  ( -31.82909658242962792, -30.00000000000000000, 285.6728570749452274 ) ) ;
#8539=DIRECTION ( 'NONE',  ( -0.000000000000000000, -1.000000000000000000, 0.000000000000000000 ) ) ;
#8543=CARTESIAN_POINT ( 'NONE',  ( -159.3442861576697283, 0.000000000000000000, -192.8974817588416499 ) ) ;
#8547=CONICAL_SURFACE ( 'NONE', #1948, 6.500000000000026645, 0.7853981633974476129 ) ;
#8552=FACE_OUTER_BOUND ( 'NONE', #6199, .T. ) ;
#8553=FACE_OUTER_BOUND ( 'NONE', #5723, .T. ) ;
#8564=ORIENTED_EDGE ( 'NONE', *, *, #4821, .F. ) ;
#8566=EDGE_LOOP ( 'NONE', ( #11429, #4164, #5895, #11645 ) ) ;
#8567=CARTESIAN_POINT ( 'NONE',  ( -287.1814104624966149, -29.00000000000000000, -23.44910453727292321 ) ) ;
#8568=EDGE_LOOP ( 'NONE', ( #3207, #449, #1312, #9233 ) ) ;
#8570=CIRCLE ( 'NONE', #481, 250.1999999999999602 ) ;
#8575=CARTESIAN_POINT ( 'NONE',  ( 0.000000000000000000, 0.000000000000000000, 0.000000000000000000 ) ) ;
#8577=EDGE_CURVE ( 'NONE', #6957, #7354, #10911, .T. ) ;
#8583=EDGE_LOOP ( 'NONE', ( #4219, #9179, #7483, #959 ) ) ;
#8586=LINE ( 'NONE', #12644, #2338 ) ;
#8587=EDGE_CURVE ( 'NONE', #7035, #9508, #4098, .T. ) ;
#8589=DIRECTION ( 'NONE',  ( 0.6368676505102708330, 0.000000000000000000, 0.7709731485165535192 ) ) ;
#8593=TOROIDAL_SURFACE ( 'NONE', #9858, 250.0000000000000000, 10.00000000000000000 ) ;
#8594=LINE ( 'NONE', #10649, #3300 ) ;
#8600=EDGE_CURVE ( 'NONE', #10757, #2690, #8966, .T. ) ;
#8602=EDGE_CURVE ( 'NONE', #11730, #2539, #8570, .T. ) ;
#8606=CARTESIAN_POINT ( 'NONE',  ( -225.1241593668336236, -29.00000000000000000, 185.9653539489990521 ) ) ;
#8609=EDGE_CURVE ( 'NONE', #2972, #564, #6874, .T. ) ;
#8610=DIRECTION ( 'NONE',  ( -0.000000000000000000, -1.000000000000000000, 0.000000000000000000 ) ) ;
#8613=CIRCLE ( 'NONE', #1801, 5.100000000000017408 ) ;
#8614=CARTESIAN_POINT ( 'NONE',  ( -31.82909658242962081, -18.00000000000000000, 285.6728570749452274 ) ) ;
#8616=ORIENTED_EDGE ( 'NONE', *, *, #4064, .F. ) ;
#8618=CONICAL_SURFACE ( 'NONE', #7085, 6.500000000000005329, 0.7853981633974547183 ) ;
#8619=AXIS2_PLACEMENT_3D ( 'NONE', #11614, #12604, #3464 ) ;
#8620=CARTESIAN_POINT ( 'NONE',  ( -225.1241593668336236, -30.00000000000000000, 185.9653539489990521 ) ) ;
#8628=VERTEX_POINT ( 'NONE', #1224 ) ;
#8638=DIRECTION ( 'NONE',  ( -0.000000000000000000, -1.000000000000000000, 0.000000000000000000 ) ) ;
#8639=CARTESIAN_POINT ( 'NONE',  ( 159.3442861576696998, 0.000000000000000000, 192.8974817588416784 ) ) ;
#8642=ORIENTED_EDGE ( 'NONE', *, *, #6698, .T. ) ;
#8643=DIRECTION ( 'NONE',  ( 0.6368676505102707219, 0.000000000000000000, 0.7709731485165536302 ) ) ;
#8644=CIRCLE ( 'NONE', #2879, 5.500000000000007994 ) ;
#8645=ORIENTED_EDGE ( 'NONE', *, *, #1828, .T. ) ;
#8648=DIRECTION ( 'NONE',  ( 0.6368676505102700558, 0.000000000000000000, 0.7709731485165541853 ) ) ;
#8650=EDGE_CURVE ( 'NONE', #4613, #1970, #3451, .T. ) ;
#8651=DIRECTION ( 'NONE',  ( -0.000000000000000000, -1.000000000000000000, 0.000000000000000000 ) ) ;
#8658=DIRECTION ( 'NONE',  ( 0.000000000000000000, 1.000000000000000000, 0.000000000000000000 ) ) ;
#8661=CARTESIAN_POINT ( 'NONE',  ( 153.9282213272189495, -18.00000000000000000, 245.7765299597151341 ) ) ;
#8671=VECTOR ( 'NONE', #1865, 1000.000000000000114 ) ;
#8674=EDGE_LOOP ( 'NONE', ( #11117, #4623, #9741, #7718 ) ) ;
#8678=CARTESIAN_POINT ( 'NONE',  ( 229.2637990951503753, -18.00000000000000000, -180.9540284836414514 ) ) ;
#8682=EDGE_CURVE ( 'NONE', #4419, #1170, #10260, .T. ) ;
#8683=ORIENTED_EDGE ( 'NONE', *, *, #9319, .T. ) ;
#8685=VERTEX_POINT ( 'NONE', #12428 ) ;
#8686=DIRECTION ( 'NONE',  ( 0.000000000000000000, 1.000000000000000000, 0.000000000000000000 ) ) ;
#8687=ORIENTED_EDGE ( 'NONE', *, *, #6407, .T. ) ;
#8690=ORIENTED_EDGE ( 'NONE', *, *, #7100, .T. ) ;
#8691=DIRECTION ( 'NONE',  ( -0.000000000000000000, -1.000000000000000000, 0.000000000000000000 ) ) ;
#8692=CARTESIAN_POINT ( 'NONE',  ( -293.0608542803120145, -28.60000000000000142, 6.485521991431944855 ) ) ;
#8697=CIRCLE ( 'NONE', #2938, 2.000000000000000444 ) ;
#8701=AXIS2_PLACEMENT_3D ( 'NONE', #12814, #8686, #367 ) ;
#8709=CONICAL_SURFACE ( 'NONE', #11284, 304.0000000000000000, 0.7853981633974207455 ) ;
#8712=DIRECTION ( 'NONE',  ( -0.000000000000000000, -1.000000000000000000, 0.000000000000000000 ) ) ;
#8719=ADVANCED_FACE ( 'NONE', ( #424 ), #10489, .F. ) ;
#8725=EDGE_LOOP ( 'NONE', ( #1594, #6814 ) ) ;
#8729=DIRECTION ( 'NONE',  ( -0.6368676505102689456, 0.000000000000000000, -0.7709731485165549625 ) ) ;
#8734=CARTESIAN_POINT ( 'NONE',  ( 294.8238222686200061, -30.00000000000000000, 32.70078231946946090 ) ) ;
#8741=ORIENTED_EDGE ( 'NONE', *, *, #9805, .F. ) ;
#8742=ORIENTED_EDGE ( 'NONE', *, *, #6649, .T. ) ;
#8745=EDGE_CURVE ( 'NONE', #11239, #11433, #1765, .T. ) ;
#8752=VERTEX_POINT ( 'NONE', #10491 ) ;
#8753=DIRECTION ( 'NONE',  ( -0.4503334343941818307, -0.7071067811865080488, -0.5451603414288285210 ) ) ;
#8756=CIRCLE ( 'NONE', #40, 254.1999999999999886 ) ;
#8769=CARTESIAN_POINT ( 'NONE',  ( -159.3442861576696998, 11.79660968244693997, -192.8974817588416784 ) ) ;
#8773=ORIENTED_EDGE ( 'NONE', *, *, #12004, .T. ) ;
#8774=AXIS2_PLACEMENT_3D ( 'NONE', #3529, #7539, #1108 ) ;
#8775=LINE ( 'NONE', #3709, #10033 ) ;
#8783=CARTESIAN_POINT ( 'NONE',  ( -0.000000000000000000, -21.50000000000000000, 0.000000000000000000 ) ) ;
#8785=AXIS2_PLACEMENT_3D ( 'NONE', #1102, #6111, #5240 ) ;
#8786=CARTESIAN_POINT ( 'NONE',  ( -165.3358371128624924, 2.772967769358929857, -200.1506762031210371 ) ) ;
#8787=ORIENTED_EDGE ( 'NONE', *, *, #5179, .T. ) ;
#8789=DIRECTION ( 'NONE',  ( -0.000000000000000000, -1.000000000000000000, 0.000000000000000000 ) ) ;
#8794=DIRECTION ( 'NONE',  ( -0.000000000000000000, -1.000000000000000000, 0.000000000000000000 ) ) ;
#8802=VECTOR ( 'NONE', #2901, 1000.000000000000000 ) ;
#8812=EDGE_CURVE ( 'NONE', #11730, #7406, #226, .T. ) ;
#8820=VERTEX_POINT ( 'NONE', #8678 ) ;
#8822=AXIS2_PLACEMENT_3D ( 'NONE', #148, #12532, #5405 ) ;
#8824=ORIENTED_EDGE ( 'NONE', *, *, #6081, .T. ) ;
#8836=ADVANCED_FACE ( 'NONE', ( #6693 ), #10692, .F. ) ;
#8837=ORIENTED_EDGE ( 'NONE', *, *, #2881, .F. ) ;
#8840=ORIENTED_EDGE ( 'NONE', *, *, #9525, .T. ) ;
#8856=ADVANCED_FACE ( 'NONE', ( #12878 ), #12403, .F. ) ;
#8857=ORIENTED_EDGE ( 'NONE', *, *, #3823, .T. ) ;
#8873=DIRECTION ( 'NONE',  ( -0.000000000000000000, -1.000000000000000000, 0.000000000000000000 ) ) ;
#8874=DIRECTION ( 'NONE',  ( -0.000000000000000000, -1.000000000000000000, 0.000000000000000000 ) ) ;
#8877=DIRECTION ( 'NONE',  ( 0.000000000000000000, 1.000000000000000000, 0.000000000000000000 ) ) ;
#8881=ORIENTED_EDGE ( 'NONE', *, *, #5666, .T. ) ;
#8883=ADVANCED_FACE ( 'NONE', ( #9674 ), #268, .F. ) ;
#8884=CYLINDRICAL_SURFACE ( 'NONE', #5722, 5.100000000000017408 ) ;
#8892=CIRCLE ( 'NONE', #3001, 5.499999999999986677 ) ;
#8899=DIRECTION ( 'NONE',  ( 0.6368676505102707219, 0.000000000000000000, 0.7709731485165536302 ) ) ;
#8901=ORIENTED_EDGE ( 'NONE', *, *, #8106, .T. ) ;
#8906=CARTESIAN_POINT ( 'NONE',  ( -0.000000000000000000, -25.00000000000000000, 0.000000000000000000 ) ) ;
#8909=ADVANCED_FACE ( 'NONE', ( #2606 ), #10615, .F. ) ;
#8924=VECTOR ( 'NONE', #10992, 1000.000000000000114 ) ;
#8926=ORIENTED_EDGE ( 'NONE', *, *, #12032, .T. ) ;
#8928=EDGE_CURVE ( 'NONE', #10624, #10245, #7818, .T. ) ;
#8929=CARTESIAN_POINT ( 'NONE',  ( 171.9542656377731191, -18.00000000000000000, 208.1627500994694628 ) ) ;
#8932=TOROIDAL_SURFACE ( 'NONE', #12747, 258.5000000000000000, 2.500000000000035083 ) ;
#8933=CARTESIAN_POINT ( 'NONE',  ( -294.8238222686198355, -30.00000000000000000, -32.70078231947154279 ) ) ;
#8936=AXIS2_PLACEMENT_3D ( 'NONE', #2694, #8712, #5779 ) ;
#8943=CARTESIAN_POINT ( 'NONE',  ( -220.9845196385168435, -30.00000000000000000, 190.9766794143566528 ) ) ;
#8944=EDGE_LOOP ( 'NONE', ( #12803, #9219, #11764, #2155 ) ) ;
#8945=VERTEX_POINT ( 'NONE', #4602 ) ;
#8946=AXIS2_PLACEMENT_3D ( 'NONE', #8279, #9206, #3323 ) ;
#8947=CARTESIAN_POINT ( 'NONE',  ( 228.6269314446401211, -30.00000000000000000, -181.7250016321579835 ) ) ;
#8961=AXIS2_PLACEMENT_3D ( 'NONE', #5671, #10800, #4659 ) ;
#8966=LINE ( 'NONE', #11023, #1540 ) ;
#8967=DIRECTION ( 'NONE',  ( -0.000000000000000000, -1.000000000000000000, 0.000000000000000000 ) ) ;
#8969=CARTESIAN_POINT ( 'NONE',  ( 225.1241593668336236, -19.00000000000000000, -185.9653539489990521 ) ) ;
#8973=TOROIDAL_SURFACE ( 'NONE', #9596, 250.0000000000000000, 10.00000000000000000 ) ;
#8975=CARTESIAN_POINT ( 'NONE',  ( 185.9653539490014111, -30.00000000000000000, 225.1241593668316625 ) ) ;
#8984=EDGE_LOOP ( 'NONE', ( #322, #1033, #7531, #7918 ) ) ;
#8986=ORIENTED_EDGE ( 'NONE', *, *, #9125, .F. ) ;
#8992=ORIENTED_EDGE ( 'NONE', *, *, #4996, .T. ) ;
#8993=AXIS2_PLACEMENT_3D ( 'NONE', #2063, #8141, #9133 ) ;
#9005=EDGE_CURVE ( 'NONE', #5611, #2751, #6031, .T. ) ;
#9009=ORIENTED_EDGE ( 'NONE', *, *, #9934, .T. ) ;
#9012=EDGE_CURVE ( 'NONE', #2751, #5611, #75, .T. ) ;
#9014=AXIS2_PLACEMENT_3D ( 'NONE', #5378, #321, #124 ) ;
#9018=DIRECTION ( 'NONE',  ( -0.000000000000000000, -1.000000000000000000, 0.000000000000000000 ) ) ;
#9020=AXIS2_PLACEMENT_3D ( 'NONE', #12141, #4068, #5060 ) ;
#9024=DIRECTION ( 'NONE',  ( 0.6368676505102737195, 0.000000000000000000, 0.7709731485165509657 ) ) ;
#9027=CIRCLE ( 'NONE', #12008, 6.500000000000005329 ) ;
#9028=CARTESIAN_POINT ( 'NONE',  ( -194.2446334056326123, 0.000000000000000000, -235.1468102975487682 ) ) ;
#9029=EDGE_LOOP ( 'NONE', ( #4911, #2329 ) ) ;
#9030=DIRECTION ( 'NONE',  ( -0.000000000000000000, -1.000000000000000000, 0.000000000000000000 ) ) ;
#9032=FACE_OUTER_BOUND ( 'NONE', #7500, .T. ) ;
#9036=LINE ( 'NONE', #3829, #1144 ) ;
#9038=CARTESIAN_POINT ( 'NONE',  ( 165.7021400752469731, 1.848645179581459796, 200.5941117395221340 ) ) ;
#9040=CIRCLE ( 'NONE', #104, 5.500000000000015099 ) ;
#9043=CARTESIAN_POINT ( 'NONE',  ( 0.000000000000000000, 0.000000000000000000, 0.000000000000000000 ) ) ;
#9044=LINE ( 'NONE', #5098, #11551 ) ;
#9050=CYLINDRICAL_SURFACE ( 'NONE', #11316, 250.1999999999999602 ) ;
#9052=ORIENTED_EDGE ( 'NONE', *, *, #8587, .F. ) ;
#9053=ADVANCED_FACE ( 'NONE', ( #4874 ), #8150, .F. ) ;
#9055=ORIENTED_EDGE ( 'NONE', *, *, #253, .F. ) ;
#9056=DIRECTION ( 'NONE',  ( -0.000000000000000000, -1.000000000000000000, 0.000000000000000000 ) ) ;
#9059=FACE_OUTER_BOUND ( 'NONE', #6986, .T. ) ;
#9062=CONICAL_SURFACE ( 'NONE', #9913, 6.500000000000026645, 0.7853981633974476129 ) ;
#9065=PRODUCT_DEFINITION ( 'UNKNOWN', '', #10872, #9950 ) ;
#9075=FACE_OUTER_BOUND ( 'NONE', #1301, .T. ) ;
#9078=ADVANCED_FACE ( 'NONE', ( #12018 ), #5886, .F. ) ;
#9079=FACE_OUTER_BOUND ( 'NONE', #12748, .T. ) ;
#9081=CARTESIAN_POINT ( 'NONE',  ( 225.1241593668336236, -30.00000000000000000, -185.9653539489990521 ) ) ;
#9083=ORIENTED_EDGE ( 'NONE', *, *, #5837, .F. ) ;
#9090=CARTESIAN_POINT ( 'NONE',  ( 0.000000000000000000, 0.000000000000000000, 0.000000000000000000 ) ) ;
#9097=ORIENTED_EDGE ( 'NONE', *, *, #6973, .F. ) ;
#9098=CARTESIAN_POINT ( 'NONE',  ( 287.1814104624967854, -19.00000000000000000, 23.44910453727082356 ) ) ;
#9102=CIRCLE ( 'NONE', #1866, 5.500000000000015099 ) ;
#9104=DIRECTION ( 'NONE',  ( -0.000000000000000000, -1.000000000000000000, 0.000000000000000000 ) ) ;
#9111=VERTEX_POINT ( 'NONE', #86 ) ;
#9112=FACE_OUTER_BOUND ( 'NONE', #9188, .T. ) ;
#9116=VERTEX_POINT ( 'NONE', #12074 ) ;
#9117=AXIS2_PLACEMENT_3D ( 'NONE', #5352, #9356, #5145 ) ;
#9125=EDGE_CURVE ( 'NONE', #10768, #9111, #8081, .T. ) ;
#9131=CIRCLE ( 'NONE', #1461, 6.500000000000005329 ) ;
#9133=DIRECTION ( 'NONE',  ( 0.6368676505102700558, 0.000000000000000000, 0.7709731485165541853 ) ) ;
#9138=DIRECTION ( 'NONE',  ( 0.000000000000000000, -1.000000000000000000, 0.000000000000000000 ) ) ;
#9139=CIRCLE ( 'NONE', #1900, 6.500000000000005329 ) ;
#9141=DIRECTION ( 'NONE',  ( 0.6368676505102707219, 0.000000000000000000, 0.7709731485165535192 ) ) ;
#9146=VERTEX_POINT ( 'NONE', #6148 ) ;
#9147=DIRECTION ( 'NONE',  ( 0.000000000000000000, 1.000000000000000000, 0.000000000000000000 ) ) ;
#9150=EDGE_LOOP ( 'NONE', ( #5312, #1638, #3035, #2956 ) ) ;
#9152=EDGE_CURVE ( 'NONE', #2361, #10957, #3874, .T. ) ;
#9163=DIRECTION ( 'NONE',  ( 0.6368676505102716101, 0.000000000000000000, 0.7709731485165527420 ) ) ;
#9165=AXIS2_PLACEMENT_3D ( 'NONE', #4399, #1413, #12417 ) ;
#9172=LINE ( 'NONE', #6108, #419 ) ;
#9174=ADVANCED_FACE ( 'NONE', ( #9079 ), #1075, .F. ) ;
#9175=CARTESIAN_POINT ( 'NONE',  ( -285.6731895343928613, -30.00000000000000000, 15.42881051422395622 ) ) ;
#9176=CARTESIAN_POINT ( 'NONE',  ( -159.2169126275676945, -3.061616997868385015E-14, -192.7432871291383663 ) ) ;
#9179=ORIENTED_EDGE ( 'NONE', *, *, #9803, .F. ) ;
#9188=EDGE_LOOP ( 'NONE', ( #5755, #1722, #10547, #4640 ) ) ;
#9196=FACE_OUTER_BOUND ( 'NONE', #10722, .T. ) ;
#9206=DIRECTION ( 'NONE',  ( -0.000000000000000000, -1.000000000000000000, 0.000000000000000000 ) ) ;
#9207=CARTESIAN_POINT ( 'NONE',  ( 0.000000000000000000, 19.00000000000000000, 0.000000000000000000 ) ) ;
#9213=EDGE_LOOP ( 'NONE', ( #9947, #5626 ) ) ;
#9214=CIRCLE ( 'NONE', #10707, 270.0000000000000000 ) ;
#9217=ORIENTED_EDGE ( 'NONE', *, *, #12761, .T. ) ;
#9219=ORIENTED_EDGE ( 'NONE', *, *, #12471, .F. ) ;
#9233=ORIENTED_EDGE ( 'NONE', *, *, #12084, .F. ) ;
#9234=CARTESIAN_POINT ( 'NONE',  ( 225.1241593668336236, -18.00000000000000000, -185.9653539489990521 ) ) ;
#9237=CONICAL_SURFACE ( 'NONE', #3477, 5.500000000000015099, 0.7853981633974461696 ) ;
#9239=CYLINDRICAL_SURFACE ( 'NONE', #5996, 5.100000000000003197 ) ;
#9243=DIRECTION ( 'NONE',  ( 0.6368676505102708330, 0.000000000000000000, 0.7709731485165535192 ) ) ;
#9244=CARTESIAN_POINT ( 'NONE',  ( 0.000000000000000000, 19.00000000000000000, 0.000000000000000000 ) ) ;
#9245=EDGE_CURVE ( 'NONE', #9508, #3688, #1775, .T. ) ;
#9256=CIRCLE ( 'NONE', #4558, 6.500000000000000888 ) ;
#9265=EDGE_CURVE ( 'NONE', #564, #2972, #7936, .T. ) ;
#9268=DIRECTION ( 'NONE',  ( -0.6368676505102698338, 0.000000000000000000, -0.7709731485165541853 ) ) ;
#9281=FACE_OUTER_BOUND ( 'NONE', #8142, .T. ) ;
#9290=CARTESIAN_POINT ( 'NONE',  ( -293.9524689910264215, -30.00000000000000000, 5.406159583508762800 ) ) ;
#9298=LINE ( 'NONE', #12238, #8394 ) ;
#9299=ORIENTED_EDGE ( 'NONE', *, *, #11615, .F. ) ;
#9306=CARTESIAN_POINT ( 'NONE',  ( -0.000000000000000000, -18.00000000000000000, 0.000000000000000000 ) ) ;
#9312=DIRECTION ( 'NONE',  ( 0.6368676505102707219, 0.000000000000000000, 0.7709731485165535192 ) ) ;
#9313=AXIS2_PLACEMENT_3D ( 'NONE', #4442, #10522, #8526 ) ;
#9318=VERTEX_POINT ( 'NONE', #12279 ) ;
#9319=EDGE_CURVE ( 'NONE', #2094, #7035, #1342, .T. ) ;
#9327=( NAMED_UNIT ( * ) PLANE_ANGLE_UNIT ( ) SI_UNIT ( $, .RADIAN. ) );
#9329=DIRECTION ( 'NONE',  ( 0.6368676505102716101, 0.000000000000000000, 0.7709731485165527420 ) ) ;
#9332=FACE_OUTER_BOUND ( 'NONE', #7880, .T. ) ;
#9336=CARTESIAN_POINT ( 'NONE',  ( 159.3442861576696998, -21.50000000000000000, 192.8974817588416784 ) ) ;
#9346=AXIS2_PLACEMENT_3D ( 'NONE', #5687, #11636, #2490 ) ;
#9350=VERTEX_POINT ( 'NONE', #11343 ) ;
#9351=FACE_OUTER_BOUND ( 'NONE', #8568, .T. ) ;
#9355=CIRCLE ( 'NONE', #3594, 6.500000000000005329 ) ;
#9356=DIRECTION ( 'NONE',  ( -0.000000000000000000, -1.000000000000000000, 0.000000000000000000 ) ) ;
#9363=CIRCLE ( 'NONE', #3389, 251.1999999999999886 ) ;
#9366=VERTEX_POINT ( 'NONE', #2339 ) ;
#9367=DIRECTION ( 'NONE',  ( -0.6368676505102706109, 0.000000000000000000, -0.7709731485165535192 ) ) ;
#9368=ORIENTED_EDGE ( 'NONE', *, *, #42, .F. ) ;
#9371=CARTESIAN_POINT ( 'NONE',  ( 221.6213872890270977, -30.00000000000000000, -190.2057062658400923 ) ) ;
#9374=DIRECTION ( 'NONE',  ( 0.6368676505102708330, 0.000000000000000000, 0.7709731485165535192 ) ) ;
#9379=AXIS2_PLACEMENT_3D ( 'NONE', #4435, #12579, #7383 ) ;
#9382=VERTEX_POINT ( 'NONE', #9472 ) ;
#9383=DIRECTION ( 'NONE',  ( 0.6368676505102716101, 0.000000000000000000, 0.7709731485165527420 ) ) ;
#9393=AXIS2_PLACEMENT_3D ( 'NONE', #12959, #7695, #10764 ) ;
#9396=DIRECTION ( 'NONE',  ( 0.000000000000000000, 1.000000000000000000, 0.000000000000000000 ) ) ;
#9398=DIRECTION ( 'NONE',  ( -0.000000000000000000, -1.000000000000000000, 0.000000000000000000 ) ) ;
#9420=ORIENTED_EDGE ( 'NONE', *, *, #535, .F. ) ;
#9424=FACE_BOUND ( 'NONE', #1841, .T. ) ;
#9428=CARTESIAN_POINT ( 'NONE',  ( -27.68945685411286561, -18.00000000000000000, 290.6841825403027997 ) ) ;
#9430=DIRECTION ( 'NONE',  ( -0.000000000000000000, -1.000000000000000000, 0.000000000000000000 ) ) ;
#9431=EDGE_CURVE ( 'NONE', #8298, #5214, #3868, .T. ) ;
#9434=EDGE_LOOP ( 'NONE', ( #230, #11647, #7301, #12087 ) ) ;
#9435=DIRECTION ( 'NONE',  ( 0.6368676505102707219, 0.000000000000000000, 0.7709731485165535192 ) ) ;
#9436=VERTEX_POINT ( 'NONE', #670 ) ;
#9443=CARTESIAN_POINT ( 'NONE',  ( -0.000000000000000000, -21.50000000000000000, 0.000000000000000000 ) ) ;
#9449=CIRCLE ( 'NONE', #3900, 5.500000000000015099 ) ;
#9452=CARTESIAN_POINT ( 'NONE',  ( 225.1241593668336236, -19.00000000000000000, -185.9653539489990521 ) ) ;
#9455=ORIENTED_EDGE ( 'NONE', *, *, #1524, .T. ) ;
#9459=AXIS2_PLACEMENT_3D ( 'NONE', #11542, #403, #4453 ) ;
#9466=CARTESIAN_POINT ( 'NONE',  ( 290.6841825403032544, -19.00000000000000000, 27.68945685411186730 ) ) ;
#9467=ORIENTED_EDGE ( 'NONE', *, *, #2809, .F. ) ;
#9470=FACE_OUTER_BOUND ( 'NONE', #6241, .T. ) ;
#9471=CARTESIAN_POINT ( 'NONE',  ( 159.3442861576696998, -21.50000000000000000, 192.8974817588416784 ) ) ;
#9472=CARTESIAN_POINT ( 'NONE',  ( 31.19222893192146273, -19.00000000000000000, -286.4438302234615890 ) ) ;
#9482=ORIENTED_EDGE ( 'NONE', *, *, #5328, .F. ) ;
#9483=DIRECTION ( 'NONE',  ( 0.000000000000000000, 1.000000000000000000, 0.000000000000000000 ) ) ;
#9486=EDGE_CURVE ( 'NONE', #11239, #9649, #9717, .T. ) ;
#9488=VECTOR ( 'NONE', #12881, 1000.000000000000114 ) ;
#9504=ADVANCED_FACE ( 'NONE', ( #4721 ), #2386, .F. ) ;
#9507=CARTESIAN_POINT ( 'NONE',  ( 159.9811538081800109, -30.00000000000000000, 193.6684549073582673 ) ) ;
#9508=VERTEX_POINT ( 'NONE', #9591 ) ;
#9509=CYLINDRICAL_SURFACE ( 'NONE', #614, 250.1999999999999602 ) ;
#9510=DIRECTION ( 'NONE',  ( 0.6368676505102707219, 0.000000000000000000, 0.7709731485165536302 ) ) ;
#9516=DIRECTION ( 'NONE',  ( 0.6368676505102707219, 0.000000000000000000, 0.7709731485165536302 ) ) ;
#9520=ORIENTED_EDGE ( 'NONE', *, *, #8745, .T. ) ;
#9524=DIRECTION ( 'NONE',  ( 0.6368676505102690566, 0.000000000000000000, 0.7709731485165549625 ) ) ;
#9525=EDGE_CURVE ( 'NONE', #1949, #7844, #4654, .T. ) ;
#9533=ORIENTED_EDGE ( 'NONE', *, *, #3823, .F. ) ;
#9536=DIRECTION ( 'NONE',  ( 0.6368676505102716101, 0.000000000000000000, 0.7709731485165527420 ) ) ;
#9541=DIRECTION ( 'NONE',  ( -0.000000000000000000, -1.000000000000000000, 0.000000000000000000 ) ) ;
#9543=DIRECTION ( 'NONE',  ( 0.6368676505102716101, 0.000000000000000000, 0.7709731485165527420 ) ) ;
#9545=EDGE_LOOP ( 'NONE', ( #2485, #2146, #4430, #9083 ) ) ;
#9548=AXIS2_PLACEMENT_3D ( 'NONE', #8202, #3112, #7189 ) ;
#9549=ORIENTED_EDGE ( 'NONE', *, *, #4107, .T. ) ;
#9550=ADVANCED_FACE ( 'NONE', ( #7728 ), #5140, .F. ) ;
#9555=AXIS2_PLACEMENT_3D ( 'NONE', #3449, #9398, #4581 ) ;
#9557=DIRECTION ( 'NONE',  ( -0.6368676505102706109, 0.000000000000000000, -0.7709731485165535192 ) ) ;
#9567=EDGE_CURVE ( 'NONE', #354, #10034, #4086, .T. ) ;
#9574=CARTESIAN_POINT ( 'NONE',  ( -27.68945685411286561, -29.00000000000000000, 290.6841825403027997 ) ) ;
#9575=CARTESIAN_POINT ( 'NONE',  ( 290.6841825403032544, -30.00000000000000000, 27.68945685411186730 ) ) ;
#9576=CYLINDRICAL_SURFACE ( 'NONE', #1689, 5.500000000000015099 ) ;
#9580=DIRECTION ( 'NONE',  ( 0.6368676505102716101, 0.000000000000000000, 0.7709731485165527420 ) ) ;
#9588=DIRECTION ( 'NONE',  ( 0.4503334343941817752, -0.7071067811865080488, 0.5451603414288286320 ) ) ;
#9591=CARTESIAN_POINT ( 'NONE',  ( 165.3358371128624924, 2.772967769358929857, 200.1506762031210371 ) ) ;
#9596=AXIS2_PLACEMENT_3D ( 'NONE', #9837, #12773, #5577 ) ;
#9615=LINE ( 'NONE', #2673, #616 ) ;
#9616=ORIENTED_EDGE ( 'NONE', *, *, #11939, .T. ) ;
#9629=AXIS2_PLACEMENT_3D ( 'NONE', #279, #3127, #7211 ) ;
#9631=VECTOR ( 'NONE', #2817, 1000.000000000000000 ) ;
#9638=EDGE_CURVE ( 'NONE', #11029, #10530, #9044, .T. ) ;
#9644=DIRECTION ( 'NONE',  ( -0.000000000000000000, -1.000000000000000000, 0.000000000000000000 ) ) ;
#9649=VERTEX_POINT ( 'NONE', #1977 ) ;
#9650=VECTOR ( 'NONE', #3760, 1000.000000000000000 ) ;
#9653=VERTEX_POINT ( 'NONE', #5163 ) ;
#9656=CYLINDRICAL_SURFACE ( 'NONE', #9868, 5.500000000000015099 ) ;
#9660=VECTOR ( 'NONE', #9896, 1000.000000000000000 ) ;
#9668=ORIENTED_EDGE ( 'NONE', *, *, #10293, .F. ) ;
#9669=AXIS2_PLACEMENT_3D ( 'NONE', #637, #1573, #3558 ) ;
#9670=CIRCLE ( 'NONE', #8206, 5.499999999999986677 ) ;
#9672=DIRECTION ( 'NONE',  ( 0.6368676505102716101, 0.000000000000000000, 0.7709731485165527420 ) ) ;
#9674=FACE_OUTER_BOUND ( 'NONE', #2199, .T. ) ;
#9676=CARTESIAN_POINT ( 'NONE',  ( -194.2446334056325270, -29.00000000000000000, -235.1468102975487682 ) ) ;
#9683=ORIENTED_EDGE ( 'NONE', *, *, #3286, .F. ) ;
#9686=CARTESIAN_POINT ( 'NONE',  ( 0.000000000000000000, 9.830508068689120194, 0.000000000000000000 ) ) ;
#9702=DIRECTION ( 'NONE',  ( 0.000000000000000000, 1.000000000000000000, 0.000000000000000000 ) ) ;
#9704=CARTESIAN_POINT ( 'NONE',  ( -289.8128292627096130, -30.00000000000000000, 10.41748504886635907 ) ) ;
#9708=ORIENTED_EDGE ( 'NONE', *, *, #2203, .T. ) ;
#9711=ORIENTED_EDGE ( 'NONE', *, *, #11172, .T. ) ;
#9716=DIRECTION ( 'NONE',  ( -0.6368676505102708330, 0.000000000000000000, -0.7709731485165536302 ) ) ;
#9717=LINE ( 'NONE', #8543, #11114 ) ;
#9724=VECTOR ( 'NONE', #2777, 1000.000000000000000 ) ;
#9725=EDGE_CURVE ( 'NONE', #8298, #5907, #5032, .T. ) ;
#9730=FACE_BOUND ( 'NONE', #1333, .T. ) ;
#9741=ORIENTED_EDGE ( 'NONE', *, *, #3248, .F. ) ;
#9746=DIRECTION ( 'NONE',  ( -0.000000000000000000, -1.000000000000000000, 0.000000000000000000 ) ) ;
#9752=CIRCLE ( 'NONE', #11471, 5.500000000000015099 ) ;
#9757=AXIS2_PLACEMENT_3D ( 'NONE', #12284, #93, #12418 ) ;
#9759=CIRCLE ( 'NONE', #12740, 260.1830065359559967 ) ;
#9764=CONICAL_SURFACE ( 'NONE', #413, 5.499999999999986677, 0.7853981633974461696 ) ;
#9766=CARTESIAN_POINT ( 'NONE',  ( 24.18668477630849978, -29.00000000000000000, -294.9245348571436693 ) ) ;
#9768=CARTESIAN_POINT ( 'NONE',  ( 185.9653539490014111, -30.00000000000000000, 225.1241593668316625 ) ) ;
#9769=DIRECTION ( 'NONE',  ( 0.6368676505102707219, 0.000000000000000000, 0.7709731485165535192 ) ) ;
#9772=CARTESIAN_POINT ( 'NONE',  ( 150.6801963096165764, -19.40000000000000213, 241.8445669022807181 ) ) ;
#9778=ADVANCED_FACE ( 'NONE', ( #8250 ), #6440, .F. ) ;
#9779=VECTOR ( 'NONE', #6522, 1000.000000000000000 ) ;
#9780=EDGE_LOOP ( 'NONE', ( #8741, #8143 ) ) ;
#9782=ORIENTED_EDGE ( 'NONE', *, *, #6486, .T. ) ;
#9784=DIRECTION ( 'NONE',  ( -0.000000000000000000, -1.000000000000000000, 0.000000000000000000 ) ) ;
#9785=DIRECTION ( 'NONE',  ( 0.6368676505102689456, 0.000000000000000000, 0.7709731485165549625 ) ) ;
#9791=DIRECTION ( 'NONE',  ( 0.6368676505102716101, 0.000000000000000000, 0.7709731485165527420 ) ) ;
#9793=CARTESIAN_POINT ( 'NONE',  ( 185.9653539490014111, -29.00000000000000000, 225.1241593668316625 ) ) ;
#9798=ORIENTED_EDGE ( 'NONE', *, *, #6555, .T. ) ;
#9803=EDGE_CURVE ( 'NONE', #779, #9649, #5798, .T. ) ;
#9805=EDGE_CURVE ( 'NONE', #4466, #8628, #57, .T. ) ;
#9811=ORIENTED_EDGE ( 'NONE', *, *, #5009, .F. ) ;
#9812=AXIS2_PLACEMENT_3D ( 'NONE', #11587, #11451, #8648 ) ;
#9813=EDGE_LOOP ( 'NONE', ( #9097, #12834 ) ) ;
#9817=ORIENTED_EDGE ( 'NONE', *, *, #4554, .T. ) ;
#9818=CIRCLE ( 'NONE', #8130, 6.500000000000005329 ) ;
#9824=DIRECTION ( 'NONE',  ( 0.4503334343941690632, -0.7071067811865280328, 0.5451603414288133109 ) ) ;
#9827=SHAPE_REPRESENTATION_RELATIONSHIP ( 'NONE' , 'NONE' ,  #11596, #10488 ) ;
#9829=ORIENTED_EDGE ( 'NONE', *, *, #7034, .F. ) ;
#9830=DIRECTION ( 'NONE',  ( -0.000000000000000000, -1.000000000000000000, 0.000000000000000000 ) ) ;
#9831=ORIENTED_EDGE ( 'NONE', *, *, #5061, .F. ) ;
#9837=CARTESIAN_POINT ( 'NONE',  ( -0.000000000000000000, -3.061616997868385015E-14, 0.000000000000000000 ) ) ;
#9838=DIRECTION ( 'NONE',  ( -0.000000000000000000, -1.000000000000000000, 0.000000000000000000 ) ) ;
#9851=VERTEX_POINT ( 'NONE', #8508 ) ;
#9853=ORIENTED_EDGE ( 'NONE', *, *, #6198, .F. ) ;
#9858=AXIS2_PLACEMENT_3D ( 'NONE', #12530, #2526, #4391 ) ;
#9861=ADVANCED_FACE ( 'NONE', ( #12570 ), #8618, .F. ) ;
#9868=AXIS2_PLACEMENT_3D ( 'NONE', #1465, #8539, #5529 ) ;
#9873=ORIENTED_EDGE ( 'NONE', *, *, #3273, .F. ) ;
#9875=CARTESIAN_POINT ( 'NONE',  ( 290.6841825403032544, -30.00000000000000000, 27.68945685411186730 ) ) ;
#9885=CIRCLE ( 'NONE', #6273, 5.100000000000003197 ) ;
#9891=DIRECTION ( 'NONE',  ( 0.000000000000000000, 1.000000000000000000, 0.000000000000000000 ) ) ;
#9896=DIRECTION ( 'NONE',  ( -0.000000000000000000, -1.000000000000000000, 0.000000000000000000 ) ) ;
#9906=DIRECTION ( 'NONE',  ( -0.000000000000000000, -1.000000000000000000, 0.000000000000000000 ) ) ;
#9913=AXIS2_PLACEMENT_3D ( 'NONE', #2104, #3409, #2421 ) ;
#9921=CARTESIAN_POINT ( 'NONE',  ( -0.000000000000000000, -22.00000000000000000, 0.000000000000000000 ) ) ;
#9925=CARTESIAN_POINT ( 'NONE',  ( -0.000000000000000000, -29.00000000000000000, 0.000000000000000000 ) ) ;
#9929=CARTESIAN_POINT ( 'NONE',  ( 290.6841825403032544, -30.00000000000000000, 27.68945685411186730 ) ) ;
#9932=ORIENTED_EDGE ( 'NONE', *, *, #3985, .F. ) ;
#9934=EDGE_CURVE ( 'NONE', #12435, #11682, #5632, .T. ) ;
#9945=FACE_BOUND ( 'NONE', #9029, .T. ) ;
#9947=ORIENTED_EDGE ( 'NONE', *, *, #4772, .T. ) ;
#9950=PRODUCT_DEFINITION_CONTEXT ( 'detailed design', #472, 'design' ) ;
#9954=CARTESIAN_POINT ( 'NONE',  ( 221.6213872890270977, -19.00000000000000000, -190.2057062658400923 ) ) ;
#9957=DIRECTION ( 'NONE',  ( -0.000000000000000000, -1.000000000000000000, 0.000000000000000000 ) ) ;
#9960=DIRECTION ( 'NONE',  ( -0.6368676505102706109, 0.000000000000000000, -0.7709731485165535192 ) ) ;
#9961=EDGE_CURVE ( 'NONE', #12935, #10237, #10061, .T. ) ;
#9963=ORIENTED_EDGE ( 'NONE', *, *, #2134, .T. ) ;
#9964=LINE ( 'NONE', #9098, #10723 ) ;
#9970=CARTESIAN_POINT ( 'NONE',  ( -161.8917567597108587, 0.000000000000000000, -195.9813743529078636 ) ) ;
#9971=CARTESIAN_POINT ( 'NONE',  ( -27.68945685411286561, -30.00000000000000000, 290.6841825403027997 ) ) ;
#9972=AXIS2_PLACEMENT_3D ( 'NONE', #357, #5479, #1221 ) ;
#9978=AXIS2_PLACEMENT_3D ( 'NONE', #5625, #1621, #6633 ) ;
#9984=EDGE_LOOP ( 'NONE', ( #3750, #11214, #2790, #2217 ) ) ;
#9988=VERTEX_POINT ( 'NONE', #4140 ) ;
#9989=AXIS2_PLACEMENT_3D ( 'NONE', #10249, #3178, #11324 ) ;
#9991=VERTEX_POINT ( 'NONE', #8221 ) ;
#9994=VECTOR ( 'NONE', #12023, 1000.000000000000000 ) ;
#9995=CARTESIAN_POINT ( 'NONE',  ( 150.6801963096165764, -19.40000000000000213, 241.8445669022807181 ) ) ;
#9998=EDGE_CURVE ( 'NONE', #5893, #5922, #11005, .T. ) ;
#10006=EDGE_LOOP ( 'NONE', ( #10917, #65 ) ) ;
#10016=LINE ( 'NONE', #3845, #9994 ) ;
#10019=EDGE_LOOP ( 'NONE', ( #5435, #9798, #9853, #8329 ) ) ;
#10020=ORIENTED_EDGE ( 'NONE', *, *, #6529, .F. ) ;
#10021=DIRECTION ( 'NONE',  ( -0.6368676505102707219, 0.000000000000000000, -0.7709731485165536302 ) ) ;
#10022=CARTESIAN_POINT ( 'NONE',  ( 135.8846079354933352, -28.60000000000000142, -256.1940150085812888 ) ) ;
#10031=VERTEX_POINT ( 'NONE', #8080 ) ;
#10033=VECTOR ( 'NONE', #10904, 1000.000000000000114 ) ;
#10034=VERTEX_POINT ( 'NONE', #3999 ) ;
#10036=AXIS2_PLACEMENT_3D ( 'NONE', #10645, #7774, #12906 ) ;
#10039=CARTESIAN_POINT ( 'NONE',  ( -0.000000000000000000, -29.00000000000000000, 0.000000000000000000 ) ) ;
#10049=ORIENTED_EDGE ( 'NONE', *, *, #8104, .F. ) ;
#10054=CONICAL_SURFACE ( 'NONE', #11968, 305.0000000000000000, 0.7853981633974758125 ) ;
#10061=CIRCLE ( 'NONE', #484, 5.100000000000003197 ) ;
#10063=SURFACE_SIDE_STYLE ('',( #996 ) ) ;
#10069=CARTESIAN_POINT ( 'NONE',  ( -23.54981712579610331, -30.00000000000000000, 295.6955080056604288 ) ) ;
#10072=DIRECTION ( 'NONE',  ( 0.6368676505102716101, 0.000000000000000000, 0.7709731485165527420 ) ) ;
#10076=DIRECTION ( 'NONE',  ( -0.000000000000000000, -1.000000000000000000, 0.000000000000000000 ) ) ;
#10082=VERTEX_POINT ( 'NONE', #1589 ) ;
#10083=CARTESIAN_POINT ( 'NONE',  ( 192.8974817588416784, -22.00000000000000000, -159.3442861576696998 ) ) ;
#10086=ORIENTED_EDGE ( 'NONE', *, *, #253, .T. ) ;
#10088=CYLINDRICAL_SURFACE ( 'NONE', #12946, 250.1999999999999602 ) ;
#10094=DIRECTION ( 'NONE',  ( -0.4503334343941556295, 0.7071067811865489050, -0.5451603414287969906 ) ) ;
#10097=VERTEX_POINT ( 'NONE', #10648 ) ;
#10099=EDGE_CURVE ( 'NONE', #7354, #6957, #8367, .T. ) ;
#10100=CIRCLE ( 'NONE', #5201, 6.500000000000000888 ) ;
#10102=CARTESIAN_POINT ( 'NONE',  ( -182.4625818711933221, -19.00000000000000000, -220.8838070499919013 ) ) ;
#10103=CYLINDRICAL_SURFACE ( 'NONE', #4024, 250.1999999999999602 ) ;
#10106=LINE ( 'NONE', #12045, #10526 ) ;
#10111=MECHANICAL_DESIGN_GEOMETRIC_PRESENTATION_REPRESENTATION('',(#3288),#6290);
#10126=DIRECTION ( 'NONE',  ( -0.6368676505102706109, 0.000000000000000000, -0.7709731485165535192 ) ) ;
#10127=ADVANCED_FACE ( 'NONE', ( #7344 ), #272, .F. ) ;
#10142=CARTESIAN_POINT ( 'NONE',  ( -290.6841825403030839, -30.00000000000000000, -27.68945685411394919 ) ) ;
#10144=ORIENTED_EDGE ( 'NONE', *, *, #10355, .T. ) ;
#10146=LINE ( 'NONE', #1955, #2317 ) ;
#10160=DIRECTION ( 'NONE',  ( -0.000000000000000000, -1.000000000000000000, 0.000000000000000000 ) ) ;
#10166=EDGE_LOOP ( 'NONE', ( #12079, #6113 ) ) ;
#10168=EDGE_CURVE ( 'NONE', #2838, #10530, #2805, .T. ) ;
#10186=EDGE_CURVE ( 'NONE', #11682, #7165, #10263, .T. ) ;
#10188=AXIS2_PLACEMENT_3D ( 'NONE', #2845, #6993, #5866 ) ;
#10189=AXIS2_PLACEMENT_3D ( 'NONE', #290, #7288, #11355 ) ;
#10193=CONICAL_SURFACE ( 'NONE', #11905, 5.100000000000003197, 0.7853981633974503884 ) ;
#10199=CIRCLE ( 'NONE', #12545, 6.500000000000005329 ) ;
#10208=VECTOR ( 'NONE', #6141, 1000.000000000000000 ) ;
#10212=VECTOR ( 'NONE', #9906, 1000.000000000000000 ) ;
#10213=DIRECTION ( 'NONE',  ( -0.000000000000000000, -1.000000000000000000, 0.000000000000000000 ) ) ;
#10223=ORIENTED_EDGE ( 'NONE', *, *, #2336, .F. ) ;
#10234=CARTESIAN_POINT ( 'NONE',  ( 0.000000000000000000, 9.830508068689120194, 0.000000000000000000 ) ) ;
#10237=VERTEX_POINT ( 'NONE', #5307 ) ;
#10238=DIRECTION ( 'NONE',  ( -0.000000000000000000, -1.000000000000000000, 0.000000000000000000 ) ) ;
#10240=ADVANCED_FACE ( 'NONE', ( #3787 ), #11010, .T. ) ;
#10245=VERTEX_POINT ( 'NONE', #11381 ) ;
#10246=TOROIDAL_SURFACE ( 'NONE', #4493, 258.5000000000000000, 2.500000000000035083 ) ;
#10249=CARTESIAN_POINT ( 'NONE',  ( -27.68945685411286561, -29.00000000000000000, 290.6841825403027997 ) ) ;
#10258=EDGE_LOOP ( 'NONE', ( #8342, #815, #4418, #11164 ) ) ;
#10259=ORIENTED_EDGE ( 'NONE', *, *, #11245, .F. ) ;
#10260=CIRCLE ( 'NONE', #7081, 270.0000000000000000 ) ;
#10263=CIRCLE ( 'NONE', #4089, 305.0000000000000000 ) ;
#10271=VECTOR ( 'NONE', #5950, 1000.000000000000000 ) ;
#10275=EDGE_CURVE ( 'NONE', #1858, #9146, #60, .T. ) ;
#10280=DIRECTION ( 'NONE',  ( -0.000000000000000000, -1.000000000000000000, 0.000000000000000000 ) ) ;
#10286=CONICAL_SURFACE ( 'NONE', #3470, 6.500000000000005329, 0.7853981633974617127 ) ;
#10293=EDGE_CURVE ( 'NONE', #1100, #4498, #1348, .T. ) ;
#10296=ORIENTED_EDGE ( 'NONE', *, *, #1321, .T. ) ;
#10297=DIRECTION ( 'NONE',  ( -0.000000000000000000, -1.000000000000000000, 0.000000000000000000 ) ) ;
#10305=CONICAL_SURFACE ( 'NONE', #7543, 6.500000000000000888, 0.7853981633974617127 ) ;
#10308=EDGE_CURVE ( 'NONE', #3933, #2919, #9214, .T. ) ;
#10313=ORIENTED_EDGE ( 'NONE', *, *, #4038, .T. ) ;
#10337=DIRECTION ( 'NONE',  ( -0.000000000000000000, -1.000000000000000000, 0.000000000000000000 ) ) ;
#10338=VECTOR ( 'NONE', #5343, 1000.000000000000000 ) ;
#10344=ORIENTED_EDGE ( 'NONE', *, *, #2754, .F. ) ;
#10355=EDGE_CURVE ( 'NONE', #9111, #11199, #4099, .T. ) ;
#10363=EDGE_CURVE ( 'NONE', #9436, #10637, #11987, .T. ) ;
#10371=VECTOR ( 'NONE', #2574, 1000.000000000000000 ) ;
#10373=CARTESIAN_POINT ( 'NONE',  ( -0.000000000000000000, -30.00000000000000000, 0.000000000000000000 ) ) ;
#10376=ORIENTED_EDGE ( 'NONE', *, *, #8183, .F. ) ;
#10380=EDGE_CURVE ( 'NONE', #6789, #9508, #11962, .T. ) ;
#10386=CARTESIAN_POINT ( 'NONE',  ( 0.000000000000000000, 1.848645179581460019, 0.000000000000000000 ) ) ;
#10387=ADVANCED_FACE ( 'NONE', ( #511 ), #377, .F. ) ;
#10399=CONICAL_SURFACE ( 'NONE', #11898, 250.1999999999999602, 0.7853981633974758125 ) ;
#10402=CIRCLE ( 'NONE', #9346, 5.500000000000007994 ) ;
#10403=DIRECTION ( 'NONE',  ( 0.6368676505102700558, 0.000000000000000000, 0.7709731485165541853 ) ) ;
#10413=VECTOR ( 'NONE', #1641, 1000.000000000000000 ) ;
#10415=FACE_BOUND ( 'NONE', #1745, .T. ) ;
#10418=CARTESIAN_POINT ( 'NONE',  ( -0.000000000000000000, -11.79660968244695951, 0.000000000000000000 ) ) ;
#10423=VERTEX_POINT ( 'NONE', #10440 ) ;
#10429=VECTOR ( 'NONE', #9588, 1000.000000000000000 ) ;
#10438=DIRECTION ( 'NONE',  ( 0.6368676505102708330, 0.000000000000000000, 0.7709731485165535192 ) ) ;
#10440=CARTESIAN_POINT ( 'NONE',  ( 158.0678610555357295, -18.00000000000000000, 250.7878554250727632 ) ) ;
#10441=CIRCLE ( 'NONE', #2352, 250.1999999999999602 ) ;
#10444=ORIENTED_EDGE ( 'NONE', *, *, #3871, .F. ) ;
#10445=DIRECTION ( 'NONE',  ( -0.6368676505102707219, 0.000000000000000000, -0.7709731485165535192 ) ) ;
#10455=CARTESIAN_POINT ( 'NONE',  ( 0.000000000000000000, 19.00000000000000000, 0.000000000000000000 ) ) ;
#10456=CARTESIAN_POINT ( 'NONE',  ( -289.8128292627096130, -19.40000000000000213, 10.41748504886635907 ) ) ;
#10461=CIRCLE ( 'NONE', #4702, 260.1830065359515061 ) ;
#10468=FACE_OUTER_BOUND ( 'NONE', #10258, .T. ) ;
#10472=FACE_OUTER_BOUND ( 'NONE', #4637, .T. ) ;
#10480=EDGE_CURVE ( 'NONE', #11299, #1949, #7514, .T. ) ;
#10482=EDGE_LOOP ( 'NONE', ( #1923, #10785 ) ) ;
#10483=VERTEX_POINT ( 'NONE', #4893 ) ;
#10486=CIRCLE ( 'NONE', #10690, 6.500000000000005329 ) ;
#10487=EDGE_CURVE ( 'NONE', #8469, #564, #2683, .T. ) ;
#10488=ADVANCED_BREP_SHAPE_REPRESENTATION ( '', ( #5935, #805 ), #7613 ) ;
#10489=CONICAL_SURFACE ( 'NONE', #7512, 6.500000000000005329, 0.7853981633974476129 ) ;
#10491=CARTESIAN_POINT ( 'NONE',  ( -228.6269314446401211, -19.00000000000000000, 181.7250016321579835 ) ) ;
#10496=ORIENTED_EDGE ( 'NONE', *, *, #5061, .T. ) ;
#10499=CARTESIAN_POINT ( 'NONE',  ( -0.000000000000000000, -22.00000000000000000, 0.000000000000000000 ) ) ;
#10504=DIRECTION ( 'NONE',  ( -0.6368676505102706109, 0.000000000000000000, -0.7709731485165535192 ) ) ;
#10507=CARTESIAN_POINT ( 'NONE',  ( 159.2169126275676945, -3.061616997868385015E-14, 192.7432871291383663 ) ) ;
#10514=DIRECTION ( 'NONE',  ( 0.000000000000000000, 1.000000000000000000, 0.000000000000000000 ) ) ;
#10515=ADVANCED_FACE ( 'NONE', ( #6966 ), #11134, .F. ) ;
#10522=DIRECTION ( 'NONE',  ( 0.000000000000000000, 1.000000000000000000, 0.000000000000000000 ) ) ;
#10523=DIRECTION ( 'NONE',  ( -0.000000000000000000, -1.000000000000000000, 0.000000000000000000 ) ) ;
#10526=VECTOR ( 'NONE', #5984, 1000.000000000000114 ) ;
#10527=AXIS2_PLACEMENT_3D ( 'NONE', #12707, #581, #5708 ) ;
#10529=FACE_OUTER_BOUND ( 'NONE', #6505, .T. ) ;
#10530=VERTEX_POINT ( 'NONE', #5971 ) ;
#10533=CARTESIAN_POINT ( 'NONE',  ( 290.6841825403032544, -30.00000000000000000, 27.68945685411186730 ) ) ;
#10538=EDGE_CURVE ( 'NONE', #2601, #4466, #7893, .T. ) ;
#10543=CIRCLE ( 'NONE', #2859, 304.0000000000000000 ) ;
#10544=PRODUCT_DEFINITION_SHAPE ( 'NONE', 'NONE',  #9065 ) ;
#10545=CIRCLE ( 'NONE', #10762, 250.1999999999999602 ) ;
#10547=ORIENTED_EDGE ( 'NONE', *, *, #2168, .T. ) ;
#10548=ORIENTED_EDGE ( 'NONE', *, *, #911, .F. ) ;
#10549=CARTESIAN_POINT ( 'NONE',  ( 135.8846079354933352, -19.40000000000000213, -256.1940150085812888 ) ) ;
#10550=FACE_BOUND ( 'NONE', #9213, .T. ) ;
#10557=DIRECTION ( 'NONE',  ( -0.000000000000000000, -1.000000000000000000, 0.000000000000000000 ) ) ;
#10563=DIRECTION ( 'NONE',  ( 0.6368676505102707219, 0.000000000000000000, 0.7709731485165535192 ) ) ;
#10566=DIRECTION ( 'NONE',  ( -0.000000000000000000, -1.000000000000000000, 0.000000000000000000 ) ) ;
#10569=CARTESIAN_POINT ( 'NONE',  ( -221.6213872890270977, -19.00000000000000000, 190.2057062658400923 ) ) ;
#10570=DIRECTION ( 'NONE',  ( 0.6368676505102689456, 0.000000000000000000, 0.7709731485165549625 ) ) ;
#10575=LINE ( 'NONE', #8391, #7874 ) ;
#10576=CARTESIAN_POINT ( 'NONE',  ( 135.8846079354933352, -30.00000000000000000, -256.1940150085812888 ) ) ;
#10578=AXIS2_PLACEMENT_3D ( 'NONE', #6817, #8874, #4599 ) ;
#10583=DIRECTION ( 'NONE',  ( -0.000000000000000000, -1.000000000000000000, 0.000000000000000000 ) ) ;
#10592=DIRECTION ( 'NONE',  ( -0.000000000000000000, -1.000000000000000000, 0.000000000000000000 ) ) ;
#10595=EDGE_CURVE ( 'NONE', #9991, #11029, #9449, .T. ) ;
#10602=DIRECTION ( 'NONE',  ( -0.000000000000000000, -1.000000000000000000, 0.000000000000000000 ) ) ;
#10604=ORIENTED_EDGE ( 'NONE', *, *, #161, .T. ) ;
#10606=FACE_OUTER_BOUND ( 'NONE', #5418, .T. ) ;
#10609=CONICAL_SURFACE ( 'NONE', #1251, 5.500000000000015099, 0.7853981633974461696 ) ;
#10611=CIRCLE ( 'NONE', #8490, 5.500000000000015099 ) ;
#10613=CONICAL_SURFACE ( 'NONE', #4865, 5.100000000000017408, 0.7853981633974503884 ) ;
#10615=CYLINDRICAL_SURFACE ( 'NONE', #6450, 5.100000000000017408 ) ;
#10621=VECTOR ( 'NONE', #8794, 1000.000000000000000 ) ;
#10623=CARTESIAN_POINT ( 'NONE',  ( 150.6801963096165764, -30.00000000000000000, 241.8445669022807181 ) ) ;
#10624=VERTEX_POINT ( 'NONE', #427 ) ;
#10629=AXIS2_PLACEMENT_3D ( 'NONE', #9921, #8789, #11993 ) ;
#10630=CYLINDRICAL_SURFACE ( 'NONE', #720, 305.0000000000000000 ) ;
#10631=CARTESIAN_POINT ( 'NONE',  ( -0.000000000000000000, -9.830508068730530624, 0.000000000000000000 ) ) ;
#10633=CIRCLE ( 'NONE', #8936, 270.0000000000000000 ) ;
#10635=DIRECTION ( 'NONE',  ( 1.000000000000000000, 0.000000000000000000, 0.000000000000000000 ) ) ;
#10637=VERTEX_POINT ( 'NONE', #3278 ) ;
#10645=CARTESIAN_POINT ( 'NONE',  ( 153.9282213272189495, -18.00000000000000000, 245.7765299597151341 ) ) ;
#10648=CARTESIAN_POINT ( 'NONE',  ( 182.4625818711949137, -19.00000000000000000, 220.8838070499906223 ) ) ;
#10649=CARTESIAN_POINT ( 'NONE',  ( 140.0242476638101152, -30.00000000000000000, -251.1826895432237166 ) ) ;
#10651=LINE ( 'NONE', #3644, #3074 ) ;
#10654=EDGE_LOOP ( 'NONE', ( #9817, #727, #4998, #5262 ) ) ;
#10660=DIRECTION ( 'NONE',  ( -0.000000000000000000, -1.000000000000000000, 0.000000000000000000 ) ) ;
#10667=CIRCLE ( 'NONE', #4924, 6.500000000000005329 ) ;
#10669=CARTESIAN_POINT ( 'NONE',  ( -289.8128292627096130, -19.40000000000000213, 10.41748504886635907 ) ) ;
#10674=DIRECTION ( 'NONE',  ( 0.6368676505102700558, 0.000000000000000000, 0.7709731485165541853 ) ) ;
#10675=FACE_BOUND ( 'NONE', #9813, .T. ) ;
#10684=ORIENTED_EDGE ( 'NONE', *, *, #5760, .F. ) ;
#10687=CARTESIAN_POINT ( 'NONE',  ( 190.1049936773181628, -30.00000000000000000, 230.1354848321892632 ) ) ;
#10690=AXIS2_PLACEMENT_3D ( 'NONE', #2918, #12802, #7004 ) ;
#10692=CONICAL_SURFACE ( 'NONE', #4509, 6.500000000000005329, 0.7853981633974617127 ) ;
#10699=DIRECTION ( 'NONE',  ( 0.6368676505102707219, 0.000000000000000000, 0.7709731485165535192 ) ) ;
#10704=DIRECTION ( 'NONE',  ( -0.000000000000000000, -1.000000000000000000, 0.000000000000000000 ) ) ;
#10707=AXIS2_PLACEMENT_3D ( 'NONE', #9244, #8252, #2241 ) ;
#10710=DIRECTION ( 'NONE',  ( 0.6368676505102696117, 0.000000000000000000, 0.7709731485165545184 ) ) ;
#10712=DIRECTION ( 'NONE',  ( 0.6368676505102716101, 0.000000000000000000, 0.7709731485165527420 ) ) ;
#10717=CARTESIAN_POINT ( 'NONE',  ( -290.6841825403030839, -30.00000000000000000, -27.68945685411394919 ) ) ;
#10719=DIRECTION ( 'NONE',  ( 0.6368676505102707219, 0.000000000000000000, 0.7709731485165536302 ) ) ;
#10722=EDGE_LOOP ( 'NONE', ( #4917, #6517, #4243, #5279 ) ) ;
#10723=VECTOR ( 'NONE', #10094, 1000.000000000000114 ) ;
#10725=EDGE_LOOP ( 'NONE', ( #1981, #4692, #712, #2216 ) ) ;
#10740=ORIENTED_EDGE ( 'NONE', *, *, #11991, .T. ) ;
#10744=FACE_BOUND ( 'NONE', #10958, .T. ) ;
#10754=ORIENTED_EDGE ( 'NONE', *, *, #8682, .F. ) ;
#10757=VERTEX_POINT ( 'NONE', #8495 ) ;
#10758=AXIS2_PLACEMENT_3D ( 'NONE', #689, #5752, #6626 ) ;
#10760=CARTESIAN_POINT ( 'NONE',  ( 194.2446334056325554, 0.000000000000000000, 235.1468102975488250 ) ) ;
#10762=AXIS2_PLACEMENT_3D ( 'NONE', #11432, #2288, #4096 ) ;
#10764=DIRECTION ( 'NONE',  ( -0.6368676505102707219, 0.000000000000000000, -0.7709731485165535192 ) ) ;
#10765=DIRECTION ( 'NONE',  ( 0.000000000000000000, 0.000000000000000000, 1.000000000000000000 ) ) ;
#10768=VERTEX_POINT ( 'NONE', #11694 ) ;
#10772=ORIENTED_EDGE ( 'NONE', *, *, #5816, .F. ) ;
#10773=ADVANCED_FACE ( 'NONE', ( #11563 ), #10892, .F. ) ;
#10775=FACE_OUTER_BOUND ( 'NONE', #11519, .T. ) ;
#10776=DIRECTION ( 'NONE',  ( 0.6368676505102716101, 0.000000000000000000, 0.7709731485165527420 ) ) ;
#10785=ORIENTED_EDGE ( 'NONE', *, *, #9567, .F. ) ;
#10800=DIRECTION ( 'NONE',  ( -0.000000000000000000, -1.000000000000000000, 0.000000000000000000 ) ) ;
#10801=AXIS2_PLACEMENT_3D ( 'NONE', #599, #6937, #9716 ) ;
#10804=ORIENTED_EDGE ( 'NONE', *, *, #9486, .T. ) ;
#10806=EDGE_CURVE ( 'NONE', #8298, #4613, #4672, .T. ) ;
#10813=EDGE_LOOP ( 'NONE', ( #9368, #6666, #3633, #7969 ) ) ;
#10815=ORIENTED_EDGE ( 'NONE', *, *, #10538, .T. ) ;
#10816=ORIENTED_EDGE ( 'NONE', *, *, #3248, .T. ) ;
#10817=AXIS2_PLACEMENT_3D ( 'NONE', #10549, #6753, #10674 ) ;
#10820=ORIENTED_EDGE ( 'NONE', *, *, #12302, .T. ) ;
#10839=DIRECTION ( 'NONE',  ( 0.6368676505102716101, 0.000000000000000000, 0.7709731485165527420 ) ) ;
#10846=ORIENTED_EDGE ( 'NONE', *, *, #2602, .T. ) ;
#10848=VECTOR ( 'NONE', #507, 1000.000000000000000 ) ;
#10851=EDGE_LOOP ( 'NONE', ( #7497, #9708, #1719, #9533 ) ) ;
#10853=VERTEX_POINT ( 'NONE', #9676 ) ;
#10862=ADVANCED_FACE ( 'NONE', ( #4739 ), #7734, .F. ) ;
#10869=DIRECTION ( 'NONE',  ( -0.000000000000000000, -1.000000000000000000, 0.000000000000000000 ) ) ;
#10871=ORIENTED_EDGE ( 'NONE', *, *, #2151, .F. ) ;
#10872=PRODUCT_DEFINITION_FORMATION_WITH_SPECIFIED_SOURCE ( 'ANY', '', #4464, .NOT_KNOWN. ) ;
#10876=DIRECTION ( 'NONE',  ( 0.4503334343941690632, -0.7071067811865280328, 0.5451603414288133109 ) ) ;
#10879=LINE ( 'NONE', #1755, #1402 ) ;
#10880=AXIS2_PLACEMENT_3D ( 'NONE', #9575, #3570, #648 ) ;
#10881=LINE ( 'NONE', #8933, #7605 ) ;
#10885=VERTEX_POINT ( 'NONE', #5684 ) ;
#10892=CONICAL_SURFACE ( 'NONE', #77, 6.500000000000005329, 0.7853981633974547183 ) ;
#10895=( LENGTH_UNIT ( ) NAMED_UNIT ( * ) SI_UNIT ( .MILLI., .METRE. ) );
#10898=DIRECTION ( 'NONE',  ( -0.000000000000000000, -1.000000000000000000, 0.000000000000000000 ) ) ;
#10903=AXIS2_PLACEMENT_3D ( 'NONE', #6660, #11793, #2576 ) ;
#10904=DIRECTION ( 'NONE',  ( -0.4503334343941556295, 0.7071067811865489050, -0.5451603414287969906 ) ) ;
#10906=CYLINDRICAL_SURFACE ( 'NONE', #4449, 5.500000000000007994 ) ;
#10911=CIRCLE ( 'NONE', #12194, 250.1999999999999602 ) ;
#10917=ORIENTED_EDGE ( 'NONE', *, *, #446, .T. ) ;
#10918=ORIENTED_EDGE ( 'NONE', *, *, #6060, .F. ) ;
#10922=AXIS2_PLACEMENT_3D ( 'NONE', #12832, #450, #4564 ) ;
#10925=CARTESIAN_POINT ( 'NONE',  ( -27.68945685411286561, -30.00000000000000000, 290.6841825403027997 ) ) ;
#10926=AXIS2_PLACEMENT_3D ( 'NONE', #4807, #6822, #2669 ) ;
#10934=CONICAL_SURFACE ( 'NONE', #5834, 5.500000000000007994, 0.7853981633974461696 ) ;
#10942=EDGE_CURVE ( 'NONE', #5825, #7844, #6888, .T. ) ;
#10945=ADVANCED_FACE ( 'NONE', ( #9470 ), #8593, .F. ) ;
#10949=AXIS2_PLACEMENT_3D ( 'NONE', #12992, #3981, #8058 ) ;
#10950=FACE_OUTER_BOUND ( 'NONE', #1651, .T. ) ;
#10951=ORIENTED_EDGE ( 'NONE', *, *, #2151, .T. ) ;
#10957=VERTEX_POINT ( 'NONE', #12598 ) ;
#10958=EDGE_LOOP ( 'NONE', ( #6687, #1018 ) ) ;
#10960=ORIENTED_EDGE ( 'NONE', *, *, #332, .T. ) ;
#10961=ADVANCED_FACE ( 'NONE', ( #471 ), #1405, .F. ) ;
#10963=EDGE_CURVE ( 'NONE', #3038, #7702, #4529, .T. ) ;
#10969=EDGE_LOOP ( 'NONE', ( #4548, #10989, #4345, #531 ) ) ;
#10973=ORIENTED_EDGE ( 'NONE', *, *, #4351, .F. ) ;
#10974=CIRCLE ( 'NONE', #549, 260.1830065359515061 ) ;
#10976=CARTESIAN_POINT ( 'NONE',  ( -185.9653539489998195, -18.00000000000000000, -225.1241593668329699 ) ) ;
#10983=EDGE_LOOP ( 'NONE', ( #10444, #7624, #10548, #7685 ) ) ;
#10986=ORIENTED_EDGE ( 'NONE', *, *, #2924, .T. ) ;
#10987=ORIENTED_EDGE ( 'NONE', *, *, #7614, .F. ) ;
#10989=ORIENTED_EDGE ( 'NONE', *, *, #6556, .T. ) ;
#10991=DIRECTION ( 'NONE',  ( -0.6368676505102707219, 0.000000000000000000, -0.7709731485165535192 ) ) ;
#10992=DIRECTION ( 'NONE',  ( -0.4503334343941556295, 0.7071067811865489050, -0.5451603414287969906 ) ) ;
#11001=CARTESIAN_POINT ( 'NONE',  ( -190.1049936773165996, -18.00000000000000000, -230.1354848321905706 ) ) ;
#11003=ADVANCED_FACE ( 'NONE', ( #10468 ), #9656, .F. ) ;
#11005=LINE ( 'NONE', #11277, #6235 ) ;
#11006=CARTESIAN_POINT ( 'NONE',  ( 0.000000000000000000, 20.00000000000000000, 0.000000000000000000 ) ) ;
#11010=TOROIDAL_SURFACE ( 'NONE', #10801, 252.1999999999999886, 2.000000000000000000 ) ;
#11015=ORIENTED_EDGE ( 'NONE', *, *, #5923, .T. ) ;
#11023=CARTESIAN_POINT ( 'NONE',  ( 132.6365829178909621, -19.40000000000000213, -260.1259780660157048 ) ) ;
#11025=ORIENTED_EDGE ( 'NONE', *, *, #911, .T. ) ;
#11029=VERTEX_POINT ( 'NONE', #7534 ) ;
#11030=ADVANCED_FACE ( 'NONE', ( #8408 ), #9237, .F. ) ;
#11049=ADVANCED_FACE ( 'NONE', ( #5403 ), #10934, .F. ) ;
#11052=VECTOR ( 'NONE', #3493, 1000.000000000000000 ) ;
#11057=AXIS2_PLACEMENT_3D ( 'NONE', #6090, #9147, #12283 ) ;
#11067=DIRECTION ( 'NONE',  ( 0.6368676505102707219, 0.000000000000000000, 0.7709731485165535192 ) ) ;
#11069=VERTEX_POINT ( 'NONE', #4518 ) ;
#11071=DIRECTION ( 'NONE',  ( -0.6368676505102707219, 0.000000000000000000, -0.7709731485165536302 ) ) ;
#11073=LINE ( 'NONE', #1569, #1273 ) ;
#11082=DIRECTION ( 'NONE',  ( 0.000000000000000000, 1.000000000000000000, 0.000000000000000000 ) ) ;
#11089=CARTESIAN_POINT ( 'NONE',  ( -185.9653539489998195, -19.00000000000000000, -225.1241593668329699 ) ) ;
#11092=DIRECTION ( 'NONE',  ( -0.000000000000000000, -1.000000000000000000, 0.000000000000000000 ) ) ;
#11103=FACE_OUTER_BOUND ( 'NONE', #2773, .T. ) ;
#11104=LINE ( 'NONE', #9970, #5560 ) ;
#11109=DIRECTION ( 'NONE',  ( -0.000000000000000000, -1.000000000000000000, 0.000000000000000000 ) ) ;
#11114=VECTOR ( 'NONE', #7663, 1000.000000000000000 ) ;
#11117=ORIENTED_EDGE ( 'NONE', *, *, #8577, .F. ) ;
#11127=FILL_AREA_STYLE ('',( #11931 ) ) ;
#11129=CYLINDRICAL_SURFACE ( 'NONE', #4357, 5.499999999999986677 ) ;
#11130=ADVANCED_FACE ( 'NONE', ( #12923 ), #10399, .F. ) ;
#11134=CONICAL_SURFACE ( 'NONE', #5393, 251.1999999999999886, 0.7853981633974207455 ) ;
#11136=VERTEX_POINT ( 'NONE', #9995 ) ;
#11142=AXIS2_PLACEMENT_3D ( 'NONE', #1381, #1115, #7444 ) ;
#11143=CARTESIAN_POINT ( 'NONE',  ( 27.68945685411497593, -30.00000000000000000, -290.6841825403026291 ) ) ;
#11152=DIRECTION ( 'NONE',  ( 0.000000000000000000, 1.000000000000000000, 0.000000000000000000 ) ) ;
#11153=CARTESIAN_POINT ( 'NONE',  ( 294.1869546181097235, -30.00000000000000000, 31.92980917095290749 ) ) ;
#11157=EDGE_CURVE ( 'NONE', #1858, #8515, #12859, .T. ) ;
#11161=AXIS2_PLACEMENT_3D ( 'NONE', #8661, #5662, #5114 ) ;
#11162=ORIENTED_EDGE ( 'NONE', *, *, #5981, .T. ) ;
#11164=ORIENTED_EDGE ( 'NONE', *, *, #10595, .T. ) ;
#11166=EDGE_LOOP ( 'NONE', ( #6259, #1155, #9420, #11702 ) ) ;
#11168=FACE_OUTER_BOUND ( 'NONE', #7700, .T. ) ;
#11171=EDGE_CURVE ( 'NONE', #11299, #5825, #2650, .T. ) ;
#11172=EDGE_CURVE ( 'NONE', #8752, #5508, #5797, .T. ) ;
#11177=ORIENTED_EDGE ( 'NONE', *, *, #5225, .F. ) ;
#11182=EDGE_CURVE ( 'NONE', #9146, #1858, #12736, .T. ) ;
#11189=CONICAL_SURFACE ( 'NONE', #8430, 250.1999999999999602, 0.7853981633975041232 ) ;
#11199=VERTEX_POINT ( 'NONE', #2776 ) ;
#11200=ORIENTED_EDGE ( 'NONE', *, *, #7597, .F. ) ;
#11206=DIRECTION ( 'NONE',  ( 0.6368676505102696117, 0.000000000000000000, 0.7709731485165545184 ) ) ;
#11211=FACE_OUTER_BOUND ( 'NONE', #7682, .T. ) ;
#11214=ORIENTED_EDGE ( 'NONE', *, *, #355, .F. ) ;
#11215=ORIENTED_EDGE ( 'NONE', *, *, #8183, .T. ) ;
#11217=LINE ( 'NONE', #7355, #7207 ) ;
#11218=DIRECTION ( 'NONE',  ( 0.6368676505102698338, 0.000000000000000000, 0.7709731485165541853 ) ) ;
#11221=DIRECTION ( 'NONE',  ( -0.000000000000000000, -1.000000000000000000, 0.000000000000000000 ) ) ;
#11224=ORIENTED_EDGE ( 'NONE', *, *, #6081, .F. ) ;
#11228=ORIENTED_EDGE ( 'NONE', *, *, #3172, .T. ) ;
#11229=CIRCLE ( 'NONE', #9313, 269.0000000000000000 ) ;
#11237=FACE_OUTER_BOUND ( 'NONE', #3414, .T. ) ;
#11239=VERTEX_POINT ( 'NONE', #2710 ) ;
#11241=ORIENTED_EDGE ( 'NONE', *, *, #9638, .F. ) ;
#11245=EDGE_CURVE ( 'NONE', #10853, #8685, #4438, .T. ) ;
#11247=CIRCLE ( 'NONE', #3581, 5.100000000000003197 ) ;
#11255=CARTESIAN_POINT ( 'NONE',  ( 185.9653539490014111, -30.00000000000000000, 225.1241593668316625 ) ) ;
#11258=ADVANCED_FACE ( 'NONE', ( #7923 ), #11263, .F. ) ;
#11259=DIRECTION ( 'NONE',  ( 0.000000000000000000, 1.000000000000000000, 0.000000000000000000 ) ) ;
#11263=CONICAL_SURFACE ( 'NONE', #4224, 6.500000000000000888, 0.7853981633974617127 ) ;
#11268=ORIENTED_EDGE ( 'NONE', *, *, #4351, .T. ) ;
#11277=CARTESIAN_POINT ( 'NONE',  ( 157.1762463448213225, -30.00000000000000000, 249.7084930171495500 ) ) ;
#11278=ADVANCED_FACE ( 'NONE', ( #2908 ), #11473, .F. ) ;
#11282=ORIENTED_EDGE ( 'NONE', *, *, #2556, .F. ) ;
#11284=AXIS2_PLACEMENT_3D ( 'NONE', #5370, #12500, #4422 ) ;
#11286=ORIENTED_EDGE ( 'NONE', *, *, #12761, .F. ) ;
#11299=VERTEX_POINT ( 'NONE', #6268 ) ;
#11301=DIRECTION ( 'NONE',  ( -0.000000000000000000, -1.000000000000000000, 0.000000000000000000 ) ) ;
#11308=CARTESIAN_POINT ( 'NONE',  ( -27.68945685411286561, -30.00000000000000000, 290.6841825403027997 ) ) ;
#11311=CARTESIAN_POINT ( 'NONE',  ( -185.9653539489998195, -29.00000000000000000, -225.1241593668329699 ) ) ;
#11313=ORIENTED_EDGE ( 'NONE', *, *, #6903, .T. ) ;
#11316=AXIS2_PLACEMENT_3D ( 'NONE', #668, #3976, #5857 ) ;
#11324=DIRECTION ( 'NONE',  ( 0.6368676505102696117, 0.000000000000000000, 0.7709731485165545184 ) ) ;
#11332=CIRCLE ( 'NONE', #13030, 5.500000000000007994 ) ;
#11335=AXIS2_PLACEMENT_3D ( 'NONE', #10418, #11425, #1293 ) ;
#11338=AXIS2_PLACEMENT_3D ( 'NONE', #7247, #5166, #8116 ) ;
#11340=LINE ( 'NONE', #3125, #11809 ) ;
#11343=CARTESIAN_POINT ( 'NONE',  ( -293.0608542803120145, -19.40000000000000213, 6.485521991431949296 ) ) ;
#11347=ORIENTED_EDGE ( 'NONE', *, *, #6407, .F. ) ;
#11349=DIRECTION ( 'NONE',  ( -0.6368676505102707219, 0.000000000000000000, -0.7709731485165535192 ) ) ;
#11351=EDGE_LOOP ( 'NONE', ( #11241, #7670, #1352, #11415 ) ) ;
#11353=EDGE_CURVE ( 'NONE', #4274, #10097, #7426, .T. ) ;
#11355=DIRECTION ( 'NONE',  ( 0.6368676505102707219, 0.000000000000000000, 0.7709731485165535192 ) ) ;
#11362=CIRCLE ( 'NONE', #12632, 304.0000000000000000 ) ;
#11365=VERTEX_POINT ( 'NONE', #195 ) ;
#11371=ORIENTED_EDGE ( 'NONE', *, *, #3862, .T. ) ;
#11375=DIRECTION ( 'NONE',  ( -0.000000000000000000, -1.000000000000000000, 0.000000000000000000 ) ) ;
#11378=VECTOR ( 'NONE', #7115, 1000.000000000000000 ) ;
#11379=ADVANCED_FACE ( 'NONE', ( #6066 ), #8332, .F. ) ;
#11381=CARTESIAN_POINT ( 'NONE',  ( -294.8238222686198355, -30.00000000000000000, -32.70078231947154279 ) ) ;
#11383=ORIENTED_EDGE ( 'NONE', *, *, #6529, .T. ) ;
#11384=CYLINDRICAL_SURFACE ( 'NONE', #11142, 5.500000000000015099 ) ;
#11385=ORIENTED_EDGE ( 'NONE', *, *, #11937, .F. ) ;
#11389=CIRCLE ( 'NONE', #6501, 2.000000000000000444 ) ;
#11395=CARTESIAN_POINT ( 'NONE',  ( 140.0242476638101152, -18.00000000000000000, -251.1826895432237166 ) ) ;
#11401=DIRECTION ( 'NONE',  ( 0.6368676505102707219, 0.000000000000000000, 0.7709731485165535192 ) ) ;
#11404=CIRCLE ( 'NONE', #6519, 5.500000000000015099 ) ;
#11408=DIRECTION ( 'NONE',  ( -0.7709731485165536302, 0.000000000000000000, 0.6368676505102706109 ) ) ;
#11414=CARTESIAN_POINT ( 'NONE',  ( -0.000000000000000000, -25.00000000000000000, 0.000000000000000000 ) ) ;
#11415=ORIENTED_EDGE ( 'NONE', *, *, #10168, .T. ) ;
#11422=DIRECTION ( 'NONE',  ( 0.6368676505102707219, 0.000000000000000000, 0.7709731485165535192 ) ) ;
#11425=DIRECTION ( 'NONE',  ( 0.000000000000000000, 1.000000000000000000, 0.000000000000000000 ) ) ;
#11429=ORIENTED_EDGE ( 'NONE', *, *, #1507, .F. ) ;
#11432=CARTESIAN_POINT ( 'NONE',  ( -0.000000000000000000, -25.50000000000000000, 0.000000000000000000 ) ) ;
#11433=VERTEX_POINT ( 'NONE', #4252 ) ;
#11437=LINE ( 'NONE', #2238, #5304 ) ;
#11447=AXIS2_PLACEMENT_3D ( 'NONE', #6591, #6397, #6463 ) ;
#11450=DIRECTION ( 'NONE',  ( -0.6368676505102707219, 0.000000000000000000, -0.7709731485165535192 ) ) ;
#11451=DIRECTION ( 'NONE',  ( -0.000000000000000000, -1.000000000000000000, 0.000000000000000000 ) ) ;
#11453=ORIENTED_EDGE ( 'NONE', *, *, #4996, .F. ) ;
#11456=FACE_OUTER_BOUND ( 'NONE', #9984, .T. ) ;
#11467=CARTESIAN_POINT ( 'NONE',  ( -189.4681260268063170, -30.00000000000000000, -229.3645116836740385 ) ) ;
#11471=AXIS2_PLACEMENT_3D ( 'NONE', #3567, #11783, #12643 ) ;
#11473=CONICAL_SURFACE ( 'NONE', #10188, 250.1999999999999602, 0.7853981633974758125 ) ;
#11477=DIRECTION ( 'NONE',  ( 0.6368676505102709440, 0.000000000000000000, 0.7709731485165532971 ) ) ;
#11478=AXIS2_PLACEMENT_3D ( 'NONE', #2941, #7090, #1019 ) ;
#11480=ORIENTED_EDGE ( 'NONE', *, *, #5156, .T. ) ;
#11487=CIRCLE ( 'NONE', #6168, 6.500000000000000888 ) ;
#11494=ADVANCED_FACE ( 'NONE', ( #4122 ), #2531, .T. ) ;
#11496=EDGE_CURVE ( 'NONE', #5907, #3553, #4012, .T. ) ;
#11509=DIRECTION ( 'NONE',  ( -0.6368676505102707219, 0.000000000000000000, -0.7709731485165536302 ) ) ;
#11519=EDGE_LOOP ( 'NONE', ( #8161, #920, #592, #5275 ) ) ;
#11521=FACE_OUTER_BOUND ( 'NONE', #10851, .T. ) ;
#11527=ADVANCED_FACE ( 'NONE', ( #5516 ), #5524, .F. ) ;
#11529=CARTESIAN_POINT ( 'NONE',  ( -225.1241593668336236, -30.00000000000000000, 185.9653539489990521 ) ) ;
#11536=VECTOR ( 'NONE', #7705, 1000.000000000000000 ) ;
#11541=ADVANCED_FACE ( 'NONE', ( #11456 ), #9576, .F. ) ;
#11542=CARTESIAN_POINT ( 'NONE',  ( 159.2169126275676945, -3.061616997868385015E-14, 192.7432871291383663 ) ) ;
#11551=VECTOR ( 'NONE', #3160, 1000.000000000000000 ) ;
#11555=VERTEX_POINT ( 'NONE', #11395 ) ;
#11556=FACE_OUTER_BOUND ( 'NONE', #8674, .T. ) ;
#11557=FACE_BOUND ( 'NONE', #3817, .T. ) ;
#11560=DIRECTION ( 'NONE',  ( 0.6368676505102708330, 0.000000000000000000, 0.7709731485165535192 ) ) ;
#11562=AXIS2_PLACEMENT_3D ( 'NONE', #12897, #8967, #12829 ) ;
#11563=FACE_OUTER_BOUND ( 'NONE', #3846, .T. ) ;
#11570=ORIENTED_EDGE ( 'NONE', *, *, #2205, .T. ) ;
#11573=CARTESIAN_POINT ( 'NONE',  ( 287.1814104624967854, -30.00000000000000000, 23.44910453727082356 ) ) ;
#11574=DIRECTION ( 'NONE',  ( -0.000000000000000000, -1.000000000000000000, 0.000000000000000000 ) ) ;
#11578=DIRECTION ( 'NONE',  ( -0.000000000000000000, -1.000000000000000000, 0.000000000000000000 ) ) ;
#11587=CARTESIAN_POINT ( 'NONE',  ( 135.8846079354933352, -19.40000000000000213, -256.1940150085812888 ) ) ;
#11589=EDGE_CURVE ( 'NONE', #941, #10853, #4441, .T. ) ;
#11596=SHAPE_REPRESENTATION ( 'External Heavy Duty Rotating Flange Ring', ( #805 ), #7613 ) ;
#11601=AXIS2_PLACEMENT_3D ( 'NONE', #9207, #83, #12342 ) ;
#11607=DIRECTION ( 'NONE',  ( -0.6368676505102696117, 0.000000000000000000, -0.7709731485165545184 ) ) ;
#11613=ADVANCED_FACE ( 'NONE', ( #4904 ), #2952, .F. ) ;
#11614=CARTESIAN_POINT ( 'NONE',  ( 0.000000000000000000, 11.79660968244693997, 0.000000000000000000 ) ) ;
#11615=EDGE_CURVE ( 'NONE', #9653, #12948, #9139, .T. ) ;
#11616=LINE ( 'NONE', #4531, #7038 ) ;
#11619=CARTESIAN_POINT ( 'NONE',  ( -0.000000000000000000, -29.00000000000000000, 0.000000000000000000 ) ) ;
#11622=CARTESIAN_POINT ( 'NONE',  ( -287.1814104624966149, -30.00000000000000000, -23.44910453727290545 ) ) ;
#11623=DIRECTION ( 'NONE',  ( -0.6368676505102689456, 0.000000000000000000, -0.7709731485165549625 ) ) ;
#11625=AXIS2_PLACEMENT_3D ( 'NONE', #3443, #10583, #1452 ) ;
#11631=CIRCLE ( 'NONE', #5880, 6.500000000000005329 ) ;
#11635=ORIENTED_EDGE ( 'NONE', *, *, #8459, .F. ) ;
#11636=DIRECTION ( 'NONE',  ( -0.000000000000000000, -1.000000000000000000, 0.000000000000000000 ) ) ;
#11637=ORIENTED_EDGE ( 'NONE', *, *, #6859, .T. ) ;
#11638=EDGE_LOOP ( 'NONE', ( #3832, #1268, #750, #55 ) ) ;
#11642=FACE_OUTER_BOUND ( 'NONE', #2499, .T. ) ;
#11645=ORIENTED_EDGE ( 'NONE', *, *, #3460, .F. ) ;
#11647=ORIENTED_EDGE ( 'NONE', *, *, #11661, .T. ) ;
#11654=CIRCLE ( 'NONE', #12918, 5.500000000000007994 ) ;
#11655=DIRECTION ( 'NONE',  ( -0.6368676505102707219, 0.000000000000000000, -0.7709731485165535192 ) ) ;
#11661=EDGE_CURVE ( 'NONE', #9350, #12208, #11977, .T. ) ;
#11666=CARTESIAN_POINT ( 'NONE',  ( -228.6269314446401211, -19.00000000000000000, 181.7250016321579835 ) ) ;
#11670=CARTESIAN_POINT ( 'NONE',  ( 290.6841825403032544, -30.00000000000000000, 27.68945685411186730 ) ) ;
#11672=DIRECTION ( 'NONE',  ( 0.6368676505102716101, 0.000000000000000000, 0.7709731485165527420 ) ) ;
#11682=VERTEX_POINT ( 'NONE', #5709 ) ;
#11683=DIRECTION ( 'NONE',  ( -0.6368676505102707219, 0.000000000000000000, -0.7709731485165535192 ) ) ;
#11685=VECTOR ( 'NONE', #1159, 1000.000000000000000 ) ;
#11687=EDGE_CURVE ( 'NONE', #327, #10957, #10199, .T. ) ;
#11694=CARTESIAN_POINT ( 'NONE',  ( -182.4625818711933221, -19.00000000000000000, -220.8838070499919013 ) ) ;
#11696=DIRECTION ( 'NONE',  ( -0.6368676505102707219, 0.000000000000000000, -0.7709731485165535192 ) ) ;
#11697=VERTEX_POINT ( 'NONE', #2635 ) ;
#11700=EDGE_LOOP ( 'NONE', ( #3883, #11767, #4176, #4783 ) ) ;
#11701=FACE_OUTER_BOUND ( 'NONE', #2276, .T. ) ;
#11702=ORIENTED_EDGE ( 'NONE', *, *, #11157, .F. ) ;
#11704=CIRCLE ( 'NONE', #11057, 250.7000000000000171 ) ;
#11705=DIRECTION ( 'NONE',  ( 0.6368676505102716101, 0.000000000000000000, 0.7709731485165527420 ) ) ;
#11711=EDGE_CURVE ( 'NONE', #2919, #3933, #10633, .T. ) ;
#11724=FACE_OUTER_BOUND ( 'NONE', #8583, .T. ) ;
#11726=DIRECTION ( 'NONE',  ( -0.000000000000000000, -1.000000000000000000, 0.000000000000000000 ) ) ;
#11729=CARTESIAN_POINT ( 'NONE',  ( 135.8846079354933352, -19.40000000000000213, -256.1940150085812888 ) ) ;
#11730=VERTEX_POINT ( 'NONE', #2573 ) ;
#11733=CARTESIAN_POINT ( 'NONE',  ( -193.6077657551222728, -30.00000000000000000, -234.3758371490322645 ) ) ;
#11743=CIRCLE ( 'NONE', #3639, 5.100000000000017408 ) ;
#11745=CONICAL_SURFACE ( 'NONE', #10880, 6.500000000000005329, 0.7853981633974617127 ) ;
#11753=ADVANCED_FACE ( 'NONE', ( #1848 ), #10906, .F. ) ;
#11762=DIRECTION ( 'NONE',  ( -0.000000000000000000, -1.000000000000000000, 0.000000000000000000 ) ) ;
#11764=ORIENTED_EDGE ( 'NONE', *, *, #607, .T. ) ;
#11767=ORIENTED_EDGE ( 'NONE', *, *, #11182, .F. ) ;
#11769=VECTOR ( 'NONE', #965, 1000.000000000000000 ) ;
#11778=AXIS2_PLACEMENT_3D ( 'NONE', #3264, #1409, #8415 ) ;
#11783=DIRECTION ( 'NONE',  ( -0.000000000000000000, -1.000000000000000000, 0.000000000000000000 ) ) ;
#11784=ORIENTED_EDGE ( 'NONE', *, *, #5957, .T. ) ;
#11785=ADVANCED_FACE ( 'NONE', ( #5235 ), #6047, .T. ) ;
#11786=DIRECTION ( 'NONE',  ( -0.000000000000000000, -1.000000000000000000, 0.000000000000000000 ) ) ;
#11787=DIRECTION ( 'NONE',  ( 0.000000000000000000, 1.000000000000000000, 0.000000000000000000 ) ) ;
#11788=DIRECTION ( 'NONE',  ( -0.000000000000000000, -1.000000000000000000, 0.000000000000000000 ) ) ;
#11789=CIRCLE ( 'NONE', #3897, 5.500000000000015099 ) ;
#11793=DIRECTION ( 'NONE',  ( -0.000000000000000000, -1.000000000000000000, 0.000000000000000000 ) ) ;
#11796=ORIENTED_EDGE ( 'NONE', *, *, #8812, .F. ) ;
#11797=ADVANCED_FACE ( 'NONE', ( #1911 ), #10103, .F. ) ;
#11808=DIRECTION ( 'NONE',  ( 0.6368676505102716101, 0.000000000000000000, 0.7709731485165527420 ) ) ;
#11809=VECTOR ( 'NONE', #3260, 1000.000000000000000 ) ;
#11810=DIRECTION ( 'NONE',  ( 0.6368676505102716101, 0.000000000000000000, 0.7709731485165527420 ) ) ;
#11817=VERTEX_POINT ( 'NONE', #12104 ) ;
#11819=AXIS2_PLACEMENT_3D ( 'NONE', #3053, #2124, #9329 ) ;
#11821=FACE_BOUND ( 'NONE', #12094, .T. ) ;
#11825=LINE ( 'NONE', #561, #9488 ) ;
#11827=ORIENTED_EDGE ( 'NONE', *, *, #2203, .F. ) ;
#11828=EDGE_CURVE ( 'NONE', #900, #3975, #11487, .T. ) ;
#11832=VERTEX_POINT ( 'NONE', #12043 ) ;
#11843=ORIENTED_EDGE ( 'NONE', *, *, #3460, .T. ) ;
#11845=LINE ( 'NONE', #7642, #5124 ) ;
#11859=DIRECTION ( 'NONE',  ( 0.6368676505102707219, 0.000000000000000000, 0.7709731485165536302 ) ) ;
#11867=EDGE_CURVE ( 'NONE', #9988, #6569, #9172, .T. ) ;
#11875=ORIENTED_EDGE ( 'NONE', *, *, #12888, .F. ) ;
#11878=DIRECTION ( 'NONE',  ( 0.6368676505102706109, 0.000000000000000000, 0.7709731485165535192 ) ) ;
#11882=CYLINDRICAL_SURFACE ( 'NONE', #10758, 5.499999999999986677 ) ;
#11883=ORIENTED_EDGE ( 'NONE', *, *, #7831, .T. ) ;
#11893=EDGE_CURVE ( 'NONE', #12419, #237, #9355, .T. ) ;
#11895=FACE_OUTER_BOUND ( 'NONE', #7548, .T. ) ;
#11898=AXIS2_PLACEMENT_3D ( 'NONE', #862, #1730, #3652 ) ;
#11899=ORIENTED_EDGE ( 'NONE', *, *, #3786, .F. ) ;
#11905=AXIS2_PLACEMENT_3D ( 'NONE', #11729, #12526, #7394 ) ;
#11917=CIRCLE ( 'NONE', #8946, 6.500000000000005329 ) ;
#11918=ORIENTED_EDGE ( 'NONE', *, *, #8123, .F. ) ;
#11926=DIRECTION ( 'NONE',  ( 0.6368676505102707219, 0.000000000000000000, 0.7709731485165535192 ) ) ;
#11927=DIRECTION ( 'NONE',  ( -0.6368676505102707219, 0.000000000000000000, -0.7709731485165535192 ) ) ;
#11931=FILL_AREA_STYLE_COLOUR ( '', #761 ) ;
#11937=EDGE_CURVE ( 'NONE', #5214, #3553, #3227, .T. ) ;
#11939=EDGE_CURVE ( 'NONE', #12436, #9851, #11437, .T. ) ;
#11945=DIRECTION ( 'NONE',  ( 0.000000000000000000, 1.000000000000000000, 0.000000000000000000 ) ) ;
#11954=ORIENTED_EDGE ( 'NONE', *, *, #5384, .T. ) ;
#11957=EDGE_LOOP ( 'NONE', ( #7720, #3619, #12782, #10144 ) ) ;
#11962=CIRCLE ( 'NONE', #285, 10.00000000000000178 ) ;
#11963=CARTESIAN_POINT ( 'NONE',  ( 194.2446334056325554, -19.00000000000000000, 235.1468102975488250 ) ) ;
#11964=CARTESIAN_POINT ( 'NONE',  ( -289.8128292627096130, -18.00000000000000000, 10.41748504886635907 ) ) ;
#11967=CARTESIAN_POINT ( 'NONE',  ( -289.8128292627096130, -30.00000000000000000, 10.41748504886635907 ) ) ;
#11968=AXIS2_PLACEMENT_3D ( 'NONE', #6750, #10869, #11067 ) ;
#11973=ADVANCED_FACE ( 'NONE', ( #3292 ), #8709, .T. ) ;
#11975=CARTESIAN_POINT ( 'NONE',  ( -159.3442861576697283, -29.00000000000000000, -192.8974817588416499 ) ) ;
#11976=CARTESIAN_POINT ( 'NONE',  ( 159.6627199829248411, -25.00000000000000000, 193.2829683331000012 ) ) ;
#11977=LINE ( 'NONE', #3836, #10413 ) ;
#11982=AXIS2_PLACEMENT_3D ( 'NONE', #11143, #4276, #2013 ) ;
#11987=CIRCLE ( 'NONE', #5160, 6.500000000000005329 ) ;
#11991=EDGE_CURVE ( 'NONE', #2076, #3933, #8507, .T. ) ;
#11992=VERTEX_POINT ( 'NONE', #12567 ) ;
#11993=DIRECTION ( 'NONE',  ( 0.6368676505102707219, 0.000000000000000000, 0.7709731485165535192 ) ) ;
#11998=CARTESIAN_POINT ( 'NONE',  ( -0.000000000000000000, -3.327561323230905366, 0.000000000000000000 ) ) ;
#11999=CARTESIAN_POINT ( 'NONE',  ( 286.5445428119865028, -30.00000000000000000, 22.67813138875427015 ) ) ;
#12001=AXIS2_PLACEMENT_3D ( 'NONE', #8025, #4151, #11218 ) ;
#12004=EDGE_CURVE ( 'NONE', #1170, #4419, #8089, .T. ) ;
#12008=AXIS2_PLACEMENT_3D ( 'NONE', #9234, #4161, #9163 ) ;
#12009=FACE_OUTER_BOUND ( 'NONE', #695, .T. ) ;
#12014=CONICAL_SURFACE ( 'NONE', #11601, 270.0000000000000000, 0.7853981633974476129 ) ;
#12015=EDGE_CURVE ( 'NONE', #6924, #4498, #2335, .T. ) ;
#12017=EDGE_CURVE ( 'NONE', #11365, #7406, #9363, .T. ) ;
#12018=FACE_OUTER_BOUND ( 'NONE', #5715, .T. ) ;
#12023=DIRECTION ( 'NONE',  ( -0.4503334343941562956, 0.7071067811865480168, -0.5451603414287978788 ) ) ;
#12032=EDGE_CURVE ( 'NONE', #3236, #1725, #12374, .T. ) ;
#12033=CARTESIAN_POINT ( 'NONE',  ( 31.19222893192146273, -19.00000000000000000, -286.4438302234615890 ) ) ;
#12034=EDGE_LOOP ( 'NONE', ( #4160, #110, #8564, #11796 ) ) ;
#12036=ORIENTED_EDGE ( 'NONE', *, *, #2205, .F. ) ;
#12038=ORIENTED_EDGE ( 'NONE', *, *, #10308, .F. ) ;
#12040=AXIS2_PLACEMENT_3D ( 'NONE', #2095, #6437, #9367 ) ;
#12041=CARTESIAN_POINT ( 'NONE',  ( 31.19222893192146273, -30.00000000000000000, -286.4438302234615890 ) ) ;
#12043=CARTESIAN_POINT ( 'NONE',  ( 131.7449682071765835, -30.00000000000000000, -261.2053404739389180 ) ) ;
#12045=CARTESIAN_POINT ( 'NONE',  ( 139.1326329530957082, -19.40000000000000213, -252.2620519511468729 ) ) ;
#12047=AXIS2_PLACEMENT_3D ( 'NONE', #2270, #3266, #10403 ) ;
#12049=ORIENTED_EDGE ( 'NONE', *, *, #10487, .T. ) ;
#12057=DIRECTION ( 'NONE',  ( 0.6368676505102709440, 0.000000000000000000, 0.7709731485165532971 ) ) ;
#12058=EDGE_CURVE ( 'NONE', #12948, #9653, #4663, .T. ) ;
#12062=DIRECTION ( 'NONE',  ( 0.6368676505102737195, 0.000000000000000000, 0.7709731485165509657 ) ) ;
#12064=DIRECTION ( 'NONE',  ( -0.000000000000000000, -1.000000000000000000, 0.000000000000000000 ) ) ;
#12074=CARTESIAN_POINT ( 'NONE',  ( -193.6077657551223012, -18.00000000000000000, -234.3758371490321792 ) ) ;
#12076=DIRECTION ( 'NONE',  ( 0.6368676505102716101, 0.000000000000000000, 0.7709731485165527420 ) ) ;
#12078=CIRCLE ( 'NONE', #11447, 251.8333333333380608 ) ;
#12079=ORIENTED_EDGE ( 'NONE', *, *, #8928, .F. ) ;
#12084=EDGE_CURVE ( 'NONE', #10637, #9436, #4032, .T. ) ;
#12087=ORIENTED_EDGE ( 'NONE', *, *, #11939, .F. ) ;
#12094=EDGE_LOOP ( 'NONE', ( #1095, #3003 ) ) ;
#12104=CARTESIAN_POINT ( 'NONE',  ( 159.3442861576696998, 19.00000000000000000, 192.8974817588417352 ) ) ;
#12105=CIRCLE ( 'NONE', #5938, 6.500000000000005329 ) ;
#12112=AXIS2_PLACEMENT_3D ( 'NONE', #8162, #10213, #11422 ) ;
#12121=ORIENTED_EDGE ( 'NONE', *, *, #5468, .T. ) ;
#12129=AXIS2_PLACEMENT_3D ( 'NONE', #2925, #4615, #12758 ) ;
#12140=DIRECTION ( 'NONE',  ( 0.6368676505102707219, 0.000000000000000000, 0.7709731485165535192 ) ) ;
#12141=CARTESIAN_POINT ( 'NONE',  ( -160.6180214586902650, -11.79660968244695951, -194.4394280558747710 ) ) ;
#12145=DIRECTION ( 'NONE',  ( -0.000000000000000000, -1.000000000000000000, 0.000000000000000000 ) ) ;
#12150=FACE_OUTER_BOUND ( 'NONE', #12902, .T. ) ;
#12151=EDGE_LOOP ( 'NONE', ( #11480, #10804, #8881, #10344 ) ) ;
#12155=LINE ( 'NONE', #7026, #1043 ) ;
#12156=EDGE_LOOP ( 'NONE', ( #6077, #12856, #6645, #4596 ) ) ;
#12157=DIRECTION ( 'NONE',  ( 0.6368676505102698338, 0.000000000000000000, 0.7709731485165541853 ) ) ;
#12163=ADVANCED_FACE ( 'NONE', ( #9075 ), #855, .F. ) ;
#12171=DIRECTION ( 'NONE',  ( -0.000000000000000000, -1.000000000000000000, 0.000000000000000000 ) ) ;
#12175=DIRECTION ( 'NONE',  ( -0.7709731485165534082, 0.000000000000000000, 0.6368676505102708330 ) ) ;
#12176=EDGE_CURVE ( 'NONE', #3319, #5611, #11073, .T. ) ;
#12181=CARTESIAN_POINT ( 'NONE',  ( 159.9811538081799540, 20.00000000000000000, 193.6684549073582673 ) ) ;
#12190=AXIS2_PLACEMENT_3D ( 'NONE', #142, #4192, #7333 ) ;
#12194=AXIS2_PLACEMENT_3D ( 'NONE', #1961, #4956, #2027 ) ;
#12199=CARTESIAN_POINT ( 'NONE',  ( 157.1762463448213225, -19.40000000000000213, 249.7084930171495500 ) ) ;
#12208=VERTEX_POINT ( 'NONE', #8692 ) ;
#12213=CIRCLE ( 'NONE', #2413, 6.500000000000005329 ) ;
#12216=CARTESIAN_POINT ( 'NONE',  ( -185.9653539489998195, -30.00000000000000000, -225.1241593668329699 ) ) ;
#12225=AXIS2_PLACEMENT_3D ( 'NONE', #6837, #10898, #8899 ) ;
#12232=EDGE_CURVE ( 'NONE', #8469, #5922, #1061, .T. ) ;
#12236=AXIS2_PLACEMENT_3D ( 'NONE', #11998, #8132, #2979 ) ;
#12238=CARTESIAN_POINT ( 'NONE',  ( 229.2637990951503753, -30.00000000000000000, -180.9540284836414514 ) ) ;
#12240=DIRECTION ( 'NONE',  ( -0.000000000000000000, -1.000000000000000000, 0.000000000000000000 ) ) ;
#12243=CARTESIAN_POINT ( 'NONE',  ( 135.8846079354933352, -30.00000000000000000, -256.1940150085812888 ) ) ;
#12252=AXIS2_PLACEMENT_3D ( 'NONE', #392, #1521, #526 ) ;
#12253=ORIENTED_EDGE ( 'NONE', *, *, #9805, .T. ) ;
#12259=EDGE_CURVE ( 'NONE', #11682, #8685, #6770, .T. ) ;
#12266=CARTESIAN_POINT ( 'NONE',  ( -0.000000000000000000, -18.00000000000000000, 0.000000000000000000 ) ) ;
#12268=DIRECTION ( 'NONE',  ( -0.000000000000000000, -1.000000000000000000, 0.000000000000000000 ) ) ;
#12279=CARTESIAN_POINT ( 'NONE',  ( 165.7021400752470868, -1.848645179577134812, 200.5941117395223046 ) ) ;
#12281=DIRECTION ( 'NONE',  ( 0.6368676505102696117, 0.000000000000000000, 0.7709731485165545184 ) ) ;
#12282=ORIENTED_EDGE ( 'NONE', *, *, #9431, .F. ) ;
#12283=DIRECTION ( 'NONE',  ( -0.6368676505102707219, 0.000000000000000000, -0.7709731485165535192 ) ) ;
#12284=CARTESIAN_POINT ( 'NONE',  ( 27.68945685411497593, -19.00000000000000000, -290.6841825403026291 ) ) ;
#12288=DIRECTION ( 'NONE',  ( 0.6368676505102707219, 0.000000000000000000, 0.7709731485165535192 ) ) ;
#12296=ORIENTED_EDGE ( 'NONE', *, *, #3748, .F. ) ;
#12297=DIRECTION ( 'NONE',  ( 0.6368676505102716101, 0.000000000000000000, 0.7709731485165527420 ) ) ;
#12298=ORIENTED_EDGE ( 'NONE', *, *, #12397, .F. ) ;
#12302=EDGE_CURVE ( 'NONE', #4412, #1244, #7341, .T. ) ;
#12303=DIRECTION ( 'NONE',  ( 0.6368676505102737195, 0.000000000000000000, 0.7709731485165509657 ) ) ;
#12306=CARTESIAN_POINT ( 'NONE',  ( 185.9653539490014111, -30.00000000000000000, 225.1241593668316625 ) ) ;
#12310=ORIENTED_EDGE ( 'NONE', *, *, #2638, .F. ) ;
#12312=ORIENTED_EDGE ( 'NONE', *, *, #12017, .T. ) ;
#12319=CIRCLE ( 'NONE', #6367, 304.0000000000000000 ) ;
#12321=EDGE_CURVE ( 'NONE', #6953, #8515, #11917, .T. ) ;
#12328=AXIS2_PLACEMENT_3D ( 'NONE', #6506, #12562, #10563 ) ;
#12341=CARTESIAN_POINT ( 'NONE',  ( 208.1627500994694628, 20.00000000000000000, -171.9542656377731191 ) ) ;
#12342=DIRECTION ( 'NONE',  ( 0.6368676505102708330, 0.000000000000000000, 0.7709731485165535192 ) ) ;
#12347=CARTESIAN_POINT ( 'NONE',  ( 27.68945685411497593, -30.00000000000000000, -290.6841825403026291 ) ) ;
#12349=ADVANCED_FACE ( 'NONE', ( #6281, #1208 ), #1005, .F. ) ;
#12361=DIRECTION ( 'NONE',  ( -0.6368676505102707219, 0.000000000000000000, -0.7709731485165536302 ) ) ;
#12367=CARTESIAN_POINT ( 'NONE',  ( -165.7021400752471436, -1.848645179577134812, -200.5941117395223046 ) ) ;
#12374=LINE ( 'NONE', #373, #4456 ) ;
#12397=EDGE_CURVE ( 'NONE', #4274, #9366, #2068, .T. ) ;
#12403=CONICAL_SURFACE ( 'NONE', #13035, 5.499999999999986677, 0.7853981633974461696 ) ;
#12417=DIRECTION ( 'NONE',  ( 0.6368676505102707219, 0.000000000000000000, 0.7709731485165535192 ) ) ;
#12418=DIRECTION ( 'NONE',  ( -0.6368676505102696117, 0.000000000000000000, -0.7709731485165545184 ) ) ;
#12419=VERTEX_POINT ( 'NONE', #12721 ) ;
#12420=ORIENTED_EDGE ( 'NONE', *, *, #10363, .F. ) ;
#12422=EDGE_CURVE ( 'NONE', #10097, #4274, #2120, .T. ) ;
#12428=CARTESIAN_POINT ( 'NONE',  ( 194.2446334056324986, -29.00000000000000000, 235.1468102975487966 ) ) ;
#12435=VERTEX_POINT ( 'NONE', #5465 ) ;
#12436=VERTEX_POINT ( 'NONE', #6675 ) ;
#12443=CIRCLE ( 'NONE', #741, 251.8333333333299606 ) ;
#12453=CIRCLE ( 'NONE', #955, 6.500000000000005329 ) ;
#12466=DIRECTION ( 'NONE',  ( -0.000000000000000000, -1.000000000000000000, 0.000000000000000000 ) ) ;
#12467=DIRECTION ( 'NONE',  ( -0.000000000000000000, -1.000000000000000000, 0.000000000000000000 ) ) ;
#12471=EDGE_CURVE ( 'NONE', #4062, #4661, #5969, .T. ) ;
#12473=DIRECTION ( 'NONE',  ( -0.000000000000000000, -1.000000000000000000, 0.000000000000000000 ) ) ;
#12480=ORIENTED_EDGE ( 'NONE', *, *, #9152, .F. ) ;
#12482=LINE ( 'NONE', #3274, #4017 ) ;
#12500=DIRECTION ( 'NONE',  ( 0.000000000000000000, 1.000000000000000000, 0.000000000000000000 ) ) ;
#12502=DIRECTION ( 'NONE',  ( -0.000000000000000000, -1.000000000000000000, 0.000000000000000000 ) ) ;
#12507=FACE_OUTER_BOUND ( 'NONE', #12732, .T. ) ;
#12508=AXIS2_PLACEMENT_3D ( 'NONE', #10455, #3312, #9516 ) ;
#12514=ORIENTED_EDGE ( 'NONE', *, *, #12397, .T. ) ;
#12526=DIRECTION ( 'NONE',  ( 0.000000000000000000, 1.000000000000000000, 0.000000000000000000 ) ) ;
#12529=DIRECTION ( 'NONE',  ( 0.6368676505102700558, 0.000000000000000000, 0.7709731485165541853 ) ) ;
#12530=CARTESIAN_POINT ( 'NONE',  ( -0.000000000000000000, -3.061616997868385015E-14, 0.000000000000000000 ) ) ;
#12532=DIRECTION ( 'NONE',  ( -0.000000000000000000, -1.000000000000000000, 0.000000000000000000 ) ) ;
#12536=CIRCLE ( 'NONE', #9978, 6.500000000000000888 ) ;
#12537=CARTESIAN_POINT ( 'NONE',  ( -293.9524689910264215, -18.00000000000000000, 5.406159583508754807 ) ) ;
#12545=AXIS2_PLACEMENT_3D ( 'NONE', #9768, #5647, #10712 ) ;
#12547=FACE_BOUND ( 'NONE', #1827, .T. ) ;
#12548=TOROIDAL_SURFACE ( 'NONE', #5309, 252.1999999999999886, 2.000000000000000000 ) ;
#12555=AXIS2_PLACEMENT_3D ( 'NONE', #2558, #9746, #10072 ) ;
#12560=AXIS2_PLACEMENT_3D ( 'NONE', #10576, #5576, #2311 ) ;
#12562=DIRECTION ( 'NONE',  ( -0.000000000000000000, -1.000000000000000000, 0.000000000000000000 ) ) ;
#12565=CARTESIAN_POINT ( 'NONE',  ( 0.000000000000000000, 0.000000000000000000, 0.000000000000000000 ) ) ;
#12567=CARTESIAN_POINT ( 'NONE',  ( 181.8257142206846311, -18.00000000000000000, 220.1128339014740618 ) ) ;
#12569=EDGE_CURVE ( 'NONE', #779, #11069, #5530, .T. ) ;
#12570=FACE_OUTER_BOUND ( 'NONE', #12156, .T. ) ;
#12573=DIRECTION ( 'NONE',  ( -0.000000000000000000, -1.000000000000000000, 0.000000000000000000 ) ) ;
#12575=ORIENTED_EDGE ( 'NONE', *, *, #3049, .T. ) ;
#12579=DIRECTION ( 'NONE',  ( 0.000000000000000000, 1.000000000000000000, 0.000000000000000000 ) ) ;
#12585=EDGE_CURVE ( 'NONE', #2601, #5508, #1709, .T. ) ;
#12593=LINE ( 'NONE', #11666, #8073 ) ;
#12597=CARTESIAN_POINT ( 'NONE',  ( -0.000000000000000000, -25.00000000000000000, 0.000000000000000000 ) ) ;
#12598=CARTESIAN_POINT ( 'NONE',  ( 181.8257142206846311, -30.00000000000000000, 220.1128339014740618 ) ) ;
#12604=DIRECTION ( 'NONE',  ( 0.000000000000000000, 1.000000000000000000, 0.000000000000000000 ) ) ;
#12608=AXIS2_PLACEMENT_3D ( 'NONE', #10717, #6212, #5649 ) ;
#12609=ORIENTED_EDGE ( 'NONE', *, *, #3286, .T. ) ;
#12612=CARTESIAN_POINT ( 'NONE',  ( 290.6841825403032544, -19.00000000000000000, 27.68945685411186730 ) ) ;
#12622=ORIENTED_EDGE ( 'NONE', *, *, #4011, .T. ) ;
#12626=AXIS2_PLACEMENT_3D ( 'NONE', #11006, #949, #7149 ) ;
#12629=CIRCLE ( 'NONE', #6464, 5.500000000000015099 ) ;
#12631=CARTESIAN_POINT ( 'NONE',  ( -31.19222893191935242, -30.00000000000000000, 286.4438302234617595 ) ) ;
#12632=AXIS2_PLACEMENT_3D ( 'NONE', #753, #11945, #11878 ) ;
#12636=DIRECTION ( 'NONE',  ( 0.6368676505102707219, 0.000000000000000000, 0.7709731485165535192 ) ) ;
#12643=DIRECTION ( 'NONE',  ( 0.6368676505102707219, 0.000000000000000000, 0.7709731485165535192 ) ) ;
#12644=CARTESIAN_POINT ( 'NONE',  ( 159.3442861576696998, 0.000000000000000000, 192.8974817588416784 ) ) ;
#12673=EDGE_CURVE ( 'NONE', #9146, #6953, #4787, .T. ) ;
#12678=CARTESIAN_POINT ( 'NONE',  ( -185.9653539489998195, -19.00000000000000000, -225.1241593668329699 ) ) ;
#12679=FACE_BOUND ( 'NONE', #1496, .T. ) ;
#12682=CONICAL_SURFACE ( 'NONE', #6310, 6.500000000000005329, 0.7853981633974476129 ) ;
#12686=FACE_OUTER_BOUND ( 'NONE', #3565, .T. ) ;
#12690=CARTESIAN_POINT ( 'NONE',  ( -0.000000000000000000, -3.061616997868385015E-14, 0.000000000000000000 ) ) ;
#12691=EDGE_LOOP ( 'NONE', ( #6836, #12622, #94, #3828 ) ) ;
#12692=ORIENTED_EDGE ( 'NONE', *, *, #12422, .T. ) ;
#12695=DIRECTION ( 'NONE',  ( -0.000000000000000000, -1.000000000000000000, 0.000000000000000000 ) ) ;
#12696=FACE_OUTER_BOUND ( 'NONE', #9545, .T. ) ;
#12707=CARTESIAN_POINT ( 'NONE',  ( 290.6841825403032544, -19.00000000000000000, 27.68945685411186730 ) ) ;
#12712=FACE_OUTER_BOUND ( 'NONE', #5026, .T. ) ;
#12715=EDGE_LOOP ( 'NONE', ( #8310, #8690, #1763, #3994 ) ) ;
#12717=ORIENTED_EDGE ( 'NONE', *, *, #3940, .T. ) ;
#12721=CARTESIAN_POINT ( 'NONE',  ( -293.9524689910264215, -30.00000000000000000, 5.406159583508762800 ) ) ;
#12732=EDGE_LOOP ( 'NONE', ( #12121, #3348, #4484, #12766 ) ) ;
#12734=FACE_OUTER_BOUND ( 'NONE', #6568, .T. ) ;
#12736=CIRCLE ( 'NONE', #12964, 5.499999999999986677 ) ;
#12737=CIRCLE ( 'NONE', #8701, 250.7000000000000171 ) ;
#12740=AXIS2_PLACEMENT_3D ( 'NONE', #3009, #9891, #891 ) ;
#12741=EDGE_CURVE ( 'NONE', #4661, #10245, #10881, .T. ) ;
#12747=AXIS2_PLACEMENT_3D ( 'NONE', #591, #7787, #12987 ) ;
#12748=EDGE_LOOP ( 'NONE', ( #969, #10973, #5658, #9782 ) ) ;
#12752=CARTESIAN_POINT ( 'NONE',  ( 164.6302876569049829, -3.165711975795909891E-14, 199.2965588915290880 ) ) ;
#12758=DIRECTION ( 'NONE',  ( 0.6368676505102700558, 0.000000000000000000, 0.7709731485165541853 ) ) ;
#12761=EDGE_CURVE ( 'NONE', #5214, #1970, #7926, .T. ) ;
#12766=ORIENTED_EDGE ( 'NONE', *, *, #8600, .F. ) ;
#12767=DIRECTION ( 'NONE',  ( 0.6368676505102707219, 0.000000000000000000, 0.7709731485165535192 ) ) ;
#12773=DIRECTION ( 'NONE',  ( -0.000000000000000000, -1.000000000000000000, 0.000000000000000000 ) ) ;
#12779=DIRECTION ( 'NONE',  ( 0.6368676505102709440, 0.000000000000000000, 0.7709731485165532971 ) ) ;
#12782=ORIENTED_EDGE ( 'NONE', *, *, #9125, .T. ) ;
#12793=EDGE_CURVE ( 'NONE', #3319, #11817, #6126, .T. ) ;
#12799=CARTESIAN_POINT ( 'NONE',  ( 23.54981712579821362, -30.00000000000000000, -295.6955080056602583 ) ) ;
#12802=DIRECTION ( 'NONE',  ( -0.000000000000000000, -1.000000000000000000, 0.000000000000000000 ) ) ;
#12803=ORIENTED_EDGE ( 'NONE', *, *, #12741, .F. ) ;
#12804=ORIENTED_EDGE ( 'NONE', *, *, #6795, .T. ) ;
#12807=FACE_OUTER_BOUND ( 'NONE', #10654, .T. ) ;
#12814=CARTESIAN_POINT ( 'NONE',  ( -0.000000000000000000, -22.00000000000000000, 0.000000000000000000 ) ) ;
#12816=ORIENTED_EDGE ( 'NONE', *, *, #9319, .F. ) ;
#12818=CIRCLE ( 'NONE', #8993, 5.100000000000003197 ) ;
#12829=DIRECTION ( 'NONE',  ( 0.6368676505102689456, 0.000000000000000000, 0.7709731485165549625 ) ) ;
#12831=EDGE_LOOP ( 'NONE', ( #11177, #3347, #7770, #9467 ) ) ;
#12832=CARTESIAN_POINT ( 'NONE',  ( -27.68945685411286561, -19.00000000000000000, 290.6841825403027997 ) ) ;
#12834=ORIENTED_EDGE ( 'NONE', *, *, #11893, .F. ) ;
#12841=DIRECTION ( 'NONE',  ( -0.4503334343941441942, 0.7071067811865670016, -0.5451603414287832239 ) ) ;
#12845=EDGE_CURVE ( 'NONE', #5922, #2972, #2385, .T. ) ;
#12847=CARTESIAN_POINT ( 'NONE',  ( 225.1241593668336236, -18.00000000000000000, -185.9653539489990521 ) ) ;
#12856=ORIENTED_EDGE ( 'NONE', *, *, #9152, .T. ) ;
#12858=CARTESIAN_POINT ( 'NONE',  ( -0.000000000000000000, -25.50000000000000000, 0.000000000000000000 ) ) ;
#12859=LINE ( 'NONE', #6738, #8924 ) ;
#12862=CIRCLE ( 'NONE', #1166, 6.500000000000005329 ) ;
#12863=CARTESIAN_POINT ( 'NONE',  ( 135.8846079354933352, -30.00000000000000000, -256.1940150085812888 ) ) ;
#12872=ORIENTED_EDGE ( 'NONE', *, *, #1101, .T. ) ;
#12873=EDGE_CURVE ( 'NONE', #4498, #6924, #12078, .T. ) ;
#12874=AXIS2_PLACEMENT_3D ( 'NONE', #4860, #12064, #10126 ) ;
#12875=LINE ( 'NONE', #8947, #8215 ) ;
#12876=FACE_BOUND ( 'NONE', #9780, .T. ) ;
#12878=FACE_OUTER_BOUND ( 'NONE', #5946, .T. ) ;
#12881=DIRECTION ( 'NONE',  ( -0.4503334343941556295, 0.7071067811865489050, -0.5451603414287969906 ) ) ;
#12884=ORIENTED_EDGE ( 'NONE', *, *, #5677, .F. ) ;
#12888=EDGE_CURVE ( 'NONE', #2076, #366, #11229, .T. ) ;
#12897=CARTESIAN_POINT ( 'NONE',  ( 290.6841825403032544, -29.00000000000000000, 27.68945685411186730 ) ) ;
#12901=LINE ( 'NONE', #2376, #9650 ) ;
#12902=EDGE_LOOP ( 'NONE', ( #11453, #7958, #1287, #3715 ) ) ;
#12906=DIRECTION ( 'NONE',  ( 0.6368676505102695007, 0.000000000000000000, 0.7709731485165545184 ) ) ;
#12918=AXIS2_PLACEMENT_3D ( 'NONE', #5281, #4282, #2220 ) ;
#12923=FACE_OUTER_BOUND ( 'NONE', #12034, .T. ) ;
#12925=DIRECTION ( 'NONE',  ( -0.000000000000000000, -1.000000000000000000, 0.000000000000000000 ) ) ;
#12933=CIRCLE ( 'NONE', #7191, 2.000000000000000444 ) ;
#12935=VERTEX_POINT ( 'NONE', #5852 ) ;
#12946=AXIS2_PLACEMENT_3D ( 'NONE', #9090, #8095, #3010 ) ;
#12948=VERTEX_POINT ( 'NONE', #4631 ) ;
#12950=ORIENTED_EDGE ( 'NONE', *, *, #2602, .F. ) ;
#12951=AXIS2_PLACEMENT_3D ( 'NONE', #3935, #8873, #12140 ) ;
#12955=EDGE_LOOP ( 'NONE', ( #11875, #10740, #7431, #5228 ) ) ;
#12956=TOROIDAL_SURFACE ( 'NONE', #3584, 250.0000000000000000, 10.00000000000000000 ) ;
#12959=CARTESIAN_POINT ( 'NONE',  ( -0.000000000000000000, -25.00000000000000000, 0.000000000000000000 ) ) ;
#12964=AXIS2_PLACEMENT_3D ( 'NONE', #3784, #11092, #9785 ) ;
#12965=ORIENTED_EDGE ( 'NONE', *, *, #1973, .F. ) ;
#12967=AXIS2_PLACEMENT_3D ( 'NONE', #6355, #8426, #3139 ) ;
#12976=DIRECTION ( 'NONE',  ( 0.000000000000000000, 1.000000000000000000, 0.000000000000000000 ) ) ;
#12987=DIRECTION ( 'NONE',  ( 0.6368676505102707219, 0.000000000000000000, 0.7709731485165535192 ) ) ;
#12991=EDGE_CURVE ( 'NONE', #9366, #2361, #9102, .T. ) ;
#12992=CARTESIAN_POINT ( 'NONE',  ( 0.000000000000000000, 19.00000000000000000, 0.000000000000000000 ) ) ;
#13000=DIRECTION ( 'NONE',  ( 0.6368676505102689456, 0.000000000000000000, 0.7709731485165549625 ) ) ;
#13007=DIRECTION ( 'NONE',  ( -0.000000000000000000, -1.000000000000000000, 0.000000000000000000 ) ) ;
#13009=FACE_OUTER_BOUND ( 'NONE', #415, .T. ) ;
#13021=LINE ( 'NONE', #767, #5296 ) ;
#13030=AXIS2_PLACEMENT_3D ( 'NONE', #5672, #4533, #2472 ) ;
#13035=AXIS2_PLACEMENT_3D ( 'NONE', #5819, #8877, #7677 ) ;
ENDSEC;
END-ISO-10303-21;
